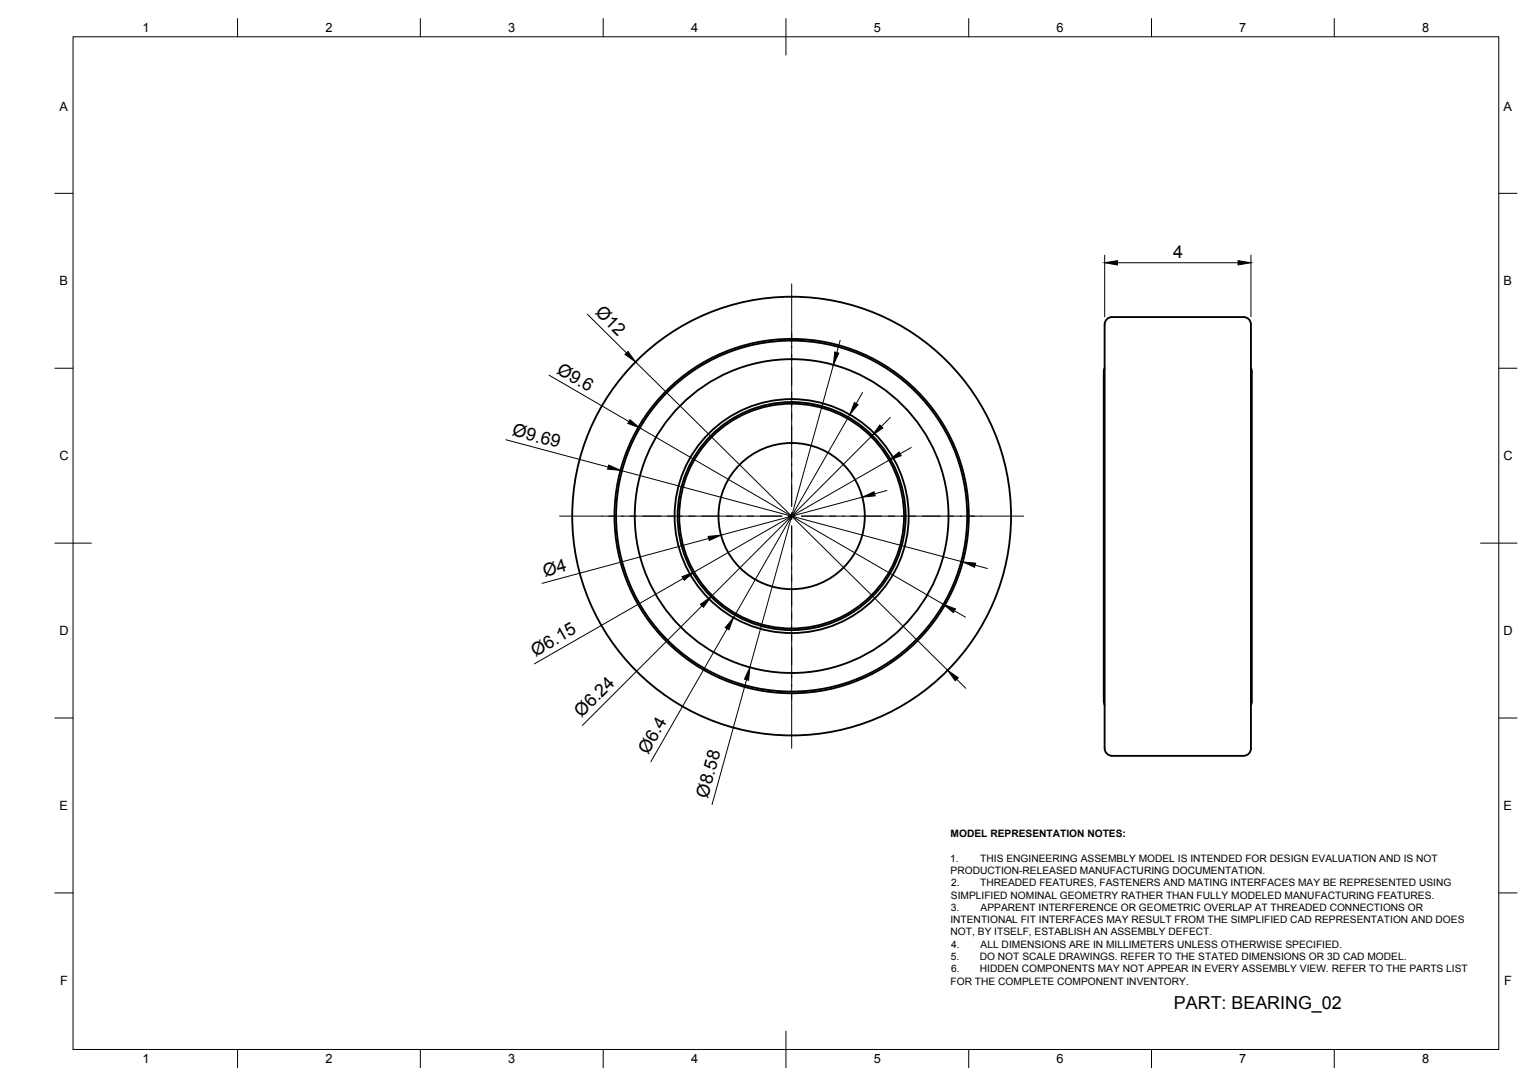
ISO-10303-21;
HEADER;
/* Generated by software containing ST-Developer
 * from STEP Tools, Inc. (www.steptools.com) 
 */

FILE_DESCRIPTION(
/* description */ (''),
/* implementation_level */ '2;1');

FILE_NAME(
/* name */ 'Bearing_02.step',
/* time_stamp */ '2026-10-04T15:18:51-07:00',
/* author */ (''),
/* organization */ (''),
/* preprocessor_version */ 'ST-DEVELOPER v20.2',
/* originating_system */ 'Autodesk Translation Framework v15.15.0.0',
/* authorisation */ '');

FILE_SCHEMA (('AUTOMOTIVE_DESIGN { 1 0 10303 214 3 1 1 }'));
ENDSEC;

DATA;
#10=MECHANICAL_DESIGN_GEOMETRIC_PRESENTATION_REPRESENTATION('',(#78,#79,#80,#81),#9891);
#59=SHAPE_REPRESENTATION_RELATIONSHIP('SRR','None',#9930,#67);
#67=ADVANCED_BREP_SHAPE_REPRESENTATION('',(#92,#93,#94,#95),#9890);
#78=STYLED_ITEM('',(#9972),#92);
#79=STYLED_ITEM('',(#9972),#93);
#80=STYLED_ITEM('',(#9972),#94);
#81=STYLED_ITEM('',(#9972),#95);
#92=MANIFOLD_SOLID_BREP('Body1',#5626);
#93=MANIFOLD_SOLID_BREP('Body2',#5627);
#94=MANIFOLD_SOLID_BREP('Body3',#5628);
#95=MANIFOLD_SOLID_BREP('Body4',#5629);
#143=FACE_BOUND('',#1063,.T.);
#144=FACE_BOUND('',#1065,.T.);
#145=FACE_BOUND('',#1067,.T.);
#146=FACE_BOUND('',#1069,.T.);
#147=FACE_BOUND('',#1081,.T.);
#148=FACE_BOUND('',#1083,.T.);
#149=FACE_BOUND('',#1085,.T.);
#150=FACE_BOUND('',#1087,.T.);
#151=FACE_BOUND('',#1101,.T.);
#152=FACE_BOUND('',#1103,.T.);
#153=FACE_BOUND('',#1105,.T.);
#154=FACE_BOUND('',#1107,.T.);
#155=FACE_BOUND('',#1109,.T.);
#156=FACE_BOUND('',#1123,.T.);
#157=FACE_BOUND('',#1125,.T.);
#158=FACE_BOUND('',#1127,.T.);
#159=FACE_BOUND('',#1129,.T.);
#160=FACE_BOUND('',#1131,.T.);
#319=PLANE('',#6244);
#320=PLANE('',#6245);
#321=PLANE('',#6246);
#322=PLANE('',#6247);
#323=PLANE('',#6277);
#324=PLANE('',#6278);
#325=PLANE('',#6279);
#326=PLANE('',#6280);
#327=PLANE('',#6317);
#328=PLANE('',#6318);
#329=PLANE('',#6319);
#330=PLANE('',#6320);
#331=PLANE('',#6321);
#332=PLANE('',#6358);
#333=PLANE('',#6359);
#334=PLANE('',#6360);
#335=PLANE('',#6361);
#336=PLANE('',#6362);
#360=TOROIDAL_SURFACE('',#6233,5.8,0.2);
#361=TOROIDAL_SURFACE('',#6239,5.8,0.2);
#362=TOROIDAL_SURFACE('',#6254,3.25741379310345,0.138976293103448);
#363=TOROIDAL_SURFACE('',#6260,3.25741379310345,0.138976293103448);
#364=TOROIDAL_SURFACE('',#6268,2.2,0.2);
#365=TOROIDAL_SURFACE('',#6274,2.2,0.2);
#366=TOROIDAL_SURFACE('',#6284,4.14313829631318,0.0900000000000005);
#367=TOROIDAL_SURFACE('',#6290,4.38370090847553,0.0200000000000002);
#368=TOROIDAL_SURFACE('',#6293,4.58,0.119999999999999);
#369=TOROIDAL_SURFACE('',#6299,4.51071796769724,0.12);
#370=TOROIDAL_SURFACE('',#6302,4.51071796769724,0.22);
#371=TOROIDAL_SURFACE('',#6308,4.58,0.219999999999999);
#372=TOROIDAL_SURFACE('',#6311,4.38370090847553,0.12);
#373=TOROIDAL_SURFACE('',#6325,4.14313829631318,0.0900000000000005);
#374=TOROIDAL_SURFACE('',#6331,4.38370090847553,0.0200000000000002);
#375=TOROIDAL_SURFACE('',#6334,4.58,0.119999999999999);
#376=TOROIDAL_SURFACE('',#6340,4.51071796769724,0.12);
#377=TOROIDAL_SURFACE('',#6343,4.51071796769724,0.22);
#378=TOROIDAL_SURFACE('',#6349,4.58,0.219999999999999);
#379=TOROIDAL_SURFACE('',#6352,4.38370090847553,0.12);
#395=CONICAL_SURFACE('',#6231,4.8,0.785398163397444);
#396=CONICAL_SURFACE('',#6242,4.845,0.785398163397444);
#397=CONICAL_SURFACE('',#6248,3.1184375,0.785398163397448);
#398=CONICAL_SURFACE('',#6266,3.0734375,0.785398163397448);
#399=CONICAL_SURFACE('',#6288,4.36638040039984,0.52359877559829);
#400=CONICAL_SURFACE('',#6297,4.57071796769724,1.04719755119659);
#401=CONICAL_SURFACE('',#6306,4.62071796769724,1.04719755119659);
#402=CONICAL_SURFACE('',#6315,4.27977786002139,0.52359877559829);
#403=CONICAL_SURFACE('',#6329,4.36638040039984,0.52359877559829);
#404=CONICAL_SURFACE('',#6338,4.57071796769724,1.04719755119659);
#405=CONICAL_SURFACE('',#6347,4.62071796769724,1.04719755119659);
#406=CONICAL_SURFACE('',#6356,4.27977786002139,0.52359877559829);
#677=FACE_OUTER_BOUND('',#1054,.T.);
#678=FACE_OUTER_BOUND('',#1055,.T.);
#679=FACE_OUTER_BOUND('',#1056,.T.);
#680=FACE_OUTER_BOUND('',#1057,.T.);
#681=FACE_OUTER_BOUND('',#1058,.T.);
#682=FACE_OUTER_BOUND('',#1059,.T.);
#683=FACE_OUTER_BOUND('',#1060,.T.);
#684=FACE_OUTER_BOUND('',#1061,.T.);
#685=FACE_OUTER_BOUND('',#1062,.T.);
#686=FACE_OUTER_BOUND('',#1064,.T.);
#687=FACE_OUTER_BOUND('',#1066,.T.);
#688=FACE_OUTER_BOUND('',#1068,.T.);
#689=FACE_OUTER_BOUND('',#1070,.T.);
#690=FACE_OUTER_BOUND('',#1071,.T.);
#691=FACE_OUTER_BOUND('',#1072,.T.);
#692=FACE_OUTER_BOUND('',#1073,.T.);
#693=FACE_OUTER_BOUND('',#1074,.T.);
#694=FACE_OUTER_BOUND('',#1075,.T.);
#695=FACE_OUTER_BOUND('',#1076,.T.);
#696=FACE_OUTER_BOUND('',#1077,.T.);
#697=FACE_OUTER_BOUND('',#1078,.T.);
#698=FACE_OUTER_BOUND('',#1079,.T.);
#699=FACE_OUTER_BOUND('',#1080,.T.);
#700=FACE_OUTER_BOUND('',#1082,.T.);
#701=FACE_OUTER_BOUND('',#1084,.T.);
#702=FACE_OUTER_BOUND('',#1086,.T.);
#703=FACE_OUTER_BOUND('',#1088,.T.);
#704=FACE_OUTER_BOUND('',#1089,.T.);
#705=FACE_OUTER_BOUND('',#1090,.T.);
#706=FACE_OUTER_BOUND('',#1091,.T.);
#707=FACE_OUTER_BOUND('',#1092,.T.);
#708=FACE_OUTER_BOUND('',#1093,.T.);
#709=FACE_OUTER_BOUND('',#1094,.T.);
#710=FACE_OUTER_BOUND('',#1095,.T.);
#711=FACE_OUTER_BOUND('',#1096,.T.);
#712=FACE_OUTER_BOUND('',#1097,.T.);
#713=FACE_OUTER_BOUND('',#1098,.T.);
#714=FACE_OUTER_BOUND('',#1099,.T.);
#715=FACE_OUTER_BOUND('',#1100,.T.);
#716=FACE_OUTER_BOUND('',#1102,.T.);
#717=FACE_OUTER_BOUND('',#1104,.T.);
#718=FACE_OUTER_BOUND('',#1106,.T.);
#719=FACE_OUTER_BOUND('',#1108,.T.);
#720=FACE_OUTER_BOUND('',#1110,.T.);
#721=FACE_OUTER_BOUND('',#1111,.T.);
#722=FACE_OUTER_BOUND('',#1112,.T.);
#723=FACE_OUTER_BOUND('',#1113,.T.);
#724=FACE_OUTER_BOUND('',#1114,.T.);
#725=FACE_OUTER_BOUND('',#1115,.T.);
#726=FACE_OUTER_BOUND('',#1116,.T.);
#727=FACE_OUTER_BOUND('',#1117,.T.);
#728=FACE_OUTER_BOUND('',#1118,.T.);
#729=FACE_OUTER_BOUND('',#1119,.T.);
#730=FACE_OUTER_BOUND('',#1120,.T.);
#731=FACE_OUTER_BOUND('',#1121,.T.);
#732=FACE_OUTER_BOUND('',#1122,.T.);
#733=FACE_OUTER_BOUND('',#1124,.T.);
#734=FACE_OUTER_BOUND('',#1126,.T.);
#735=FACE_OUTER_BOUND('',#1128,.T.);
#736=FACE_OUTER_BOUND('',#1130,.T.);
#1054=EDGE_LOOP('',(#4994,#4995,#4996,#4997));
#1055=EDGE_LOOP('',(#4998,#4999,#5000,#5001));
#1056=EDGE_LOOP('',(#5002,#5003,#5004,#5005,#5006));
#1057=EDGE_LOOP('',(#5007,#5008,#5009,#5010,#5011));
#1058=EDGE_LOOP('',(#5012,#5013,#5014,#5015));
#1059=EDGE_LOOP('',(#5016,#5017,#5018,#5019));
#1060=EDGE_LOOP('',(#5020,#5021,#5022,#5023));
#1061=EDGE_LOOP('',(#5024,#5025,#5026,#5027));
#1062=EDGE_LOOP('',(#5028));
#1063=EDGE_LOOP('',(#5029));
#1064=EDGE_LOOP('',(#5030));
#1065=EDGE_LOOP('',(#5031));
#1066=EDGE_LOOP('',(#5032));
#1067=EDGE_LOOP('',(#5033));
#1068=EDGE_LOOP('',(#5034));
#1069=EDGE_LOOP('',(#5035));
#1070=EDGE_LOOP('',(#5036,#5037,#5038,#5039,#5040));
#1071=EDGE_LOOP('',(#5041,#5042,#5043,#5044,#5045));
#1072=EDGE_LOOP('',(#5046,#5047,#5048,#5049));
#1073=EDGE_LOOP('',(#5050,#5051,#5052,#5053));
#1074=EDGE_LOOP('',(#5054,#5055,#5056,#5057));
#1075=EDGE_LOOP('',(#5058,#5059,#5060,#5061));
#1076=EDGE_LOOP('',(#5062,#5063,#5064,#5065));
#1077=EDGE_LOOP('',(#5066,#5067,#5068,#5069));
#1078=EDGE_LOOP('',(#5070,#5071,#5072,#5073));
#1079=EDGE_LOOP('',(#5074,#5075,#5076,#5077));
#1080=EDGE_LOOP('',(#5078));
#1081=EDGE_LOOP('',(#5079));
#1082=EDGE_LOOP('',(#5080));
#1083=EDGE_LOOP('',(#5081));
#1084=EDGE_LOOP('',(#5082));
#1085=EDGE_LOOP('',(#5083));
#1086=EDGE_LOOP('',(#5084));
#1087=EDGE_LOOP('',(#5085));
#1088=EDGE_LOOP('',(#5086,#5087,#5088,#5089));
#1089=EDGE_LOOP('',(#5090,#5091,#5092,#5093));
#1090=EDGE_LOOP('',(#5094,#5095,#5096,#5097));
#1091=EDGE_LOOP('',(#5098,#5099,#5100,#5101));
#1092=EDGE_LOOP('',(#5102,#5103,#5104,#5105));
#1093=EDGE_LOOP('',(#5106,#5107,#5108,#5109));
#1094=EDGE_LOOP('',(#5110,#5111,#5112,#5113));
#1095=EDGE_LOOP('',(#5114,#5115,#5116,#5117));
#1096=EDGE_LOOP('',(#5118,#5119,#5120,#5121));
#1097=EDGE_LOOP('',(#5122,#5123,#5124,#5125));
#1098=EDGE_LOOP('',(#5126,#5127,#5128,#5129));
#1099=EDGE_LOOP('',(#5130,#5131,#5132,#5133));
#1100=EDGE_LOOP('',(#5134));
#1101=EDGE_LOOP('',(#5135));
#1102=EDGE_LOOP('',(#5136));
#1103=EDGE_LOOP('',(#5137));
#1104=EDGE_LOOP('',(#5138));
#1105=EDGE_LOOP('',(#5139));
#1106=EDGE_LOOP('',(#5140));
#1107=EDGE_LOOP('',(#5141));
#1108=EDGE_LOOP('',(#5142));
#1109=EDGE_LOOP('',(#5143));
#1110=EDGE_LOOP('',(#5144,#5145,#5146,#5147));
#1111=EDGE_LOOP('',(#5148,#5149,#5150,#5151));
#1112=EDGE_LOOP('',(#5152,#5153,#5154,#5155));
#1113=EDGE_LOOP('',(#5156,#5157,#5158,#5159));
#1114=EDGE_LOOP('',(#5160,#5161,#5162,#5163));
#1115=EDGE_LOOP('',(#5164,#5165,#5166,#5167));
#1116=EDGE_LOOP('',(#5168,#5169,#5170,#5171));
#1117=EDGE_LOOP('',(#5172,#5173,#5174,#5175));
#1118=EDGE_LOOP('',(#5176,#5177,#5178,#5179));
#1119=EDGE_LOOP('',(#5180,#5181,#5182,#5183));
#1120=EDGE_LOOP('',(#5184,#5185,#5186,#5187));
#1121=EDGE_LOOP('',(#5188,#5189,#5190,#5191));
#1122=EDGE_LOOP('',(#5192));
#1123=EDGE_LOOP('',(#5193));
#1124=EDGE_LOOP('',(#5194));
#1125=EDGE_LOOP('',(#5195));
#1126=EDGE_LOOP('',(#5196));
#1127=EDGE_LOOP('',(#5197));
#1128=EDGE_LOOP('',(#5198));
#1129=EDGE_LOOP('',(#5199));
#1130=EDGE_LOOP('',(#5200));
#1131=EDGE_LOOP('',(#5201));
#1574=LINE('',#9642,#2038);
#1575=LINE('',#9648,#2039);
#1576=LINE('',#9656,#2040);
#1577=LINE('',#9660,#2041);
#1578=LINE('',#9671,#2042);
#1579=LINE('',#9678,#2043);
#1580=LINE('',#9689,#2044);
#1581=LINE('',#9694,#2045);
#1582=LINE('',#9704,#2046);
#1583=LINE('',#9714,#2047);
#1584=LINE('',#9718,#2048);
#1585=LINE('',#9728,#2049);
#1586=LINE('',#9742,#2050);
#1587=LINE('',#9753,#2051);
#1588=LINE('',#9767,#2052);
#1589=LINE('',#9781,#2053);
#1590=LINE('',#9795,#2054);
#1591=LINE('',#9805,#2055);
#1592=LINE('',#9816,#2056);
#1593=LINE('',#9830,#2057);
#1594=LINE('',#9844,#2058);
#1595=LINE('',#9858,#2059);
#2038=VECTOR('',#7821,4.8);
#2039=VECTOR('',#7828,4.872);
#2040=VECTOR('',#7837,4.8);
#2041=VECTOR('',#7842,4.8);
#2042=VECTOR('',#7857,6.);
#2043=VECTOR('',#7866,4.845);
#2044=VECTOR('',#7881,3.1184375);
#2045=VECTOR('',#7888,3.1184375);
#2046=VECTOR('',#7901,3.272);
#2047=VECTOR('',#7914,3.1184375);
#2048=VECTOR('',#7919,3.0734375);
#2049=VECTOR('',#7932,2.);
#2050=VECTOR('',#7953,3.2);
#2051=VECTOR('',#7968,4.36638040039984);
#2052=VECTOR('',#7987,4.57071796769724);
#2053=VECTOR('',#8006,4.62071796769724);
#2054=VECTOR('',#8025,4.27977786002139);
#2055=VECTOR('',#8040,3.2);
#2056=VECTOR('',#8055,4.36638040039984);
#2057=VECTOR('',#8074,4.57071796769724);
#2058=VECTOR('',#8093,4.62071796769724);
#2059=VECTOR('',#8112,4.27977786002139);
#2283=CIRCLE('',#6222,4.8);
#2284=CIRCLE('',#6223,4.8);
#2285=CIRCLE('',#6225,4.872);
#2286=CIRCLE('',#6226,4.872);
#2287=CIRCLE('',#6228,4.8);
#2288=CIRCLE('',#6229,4.8);
#2289=CIRCLE('',#6230,4.8);
#2290=CIRCLE('',#6232,4.845);
#2291=CIRCLE('',#6234,6.);
#2292=CIRCLE('',#6235,0.2);
#2293=CIRCLE('',#6236,5.8);
#2294=CIRCLE('',#6238,6.);
#2295=CIRCLE('',#6240,5.8);
#2296=CIRCLE('',#6241,0.2);
#2297=CIRCLE('',#6243,4.845);
#2298=CIRCLE('',#6249,3.1184375);
#2299=CIRCLE('',#6250,3.0734375);
#2300=CIRCLE('',#6251,3.1184375);
#2301=CIRCLE('',#6253,3.1184375);
#2302=CIRCLE('',#6255,0.138976293103448);
#2303=CIRCLE('',#6256,3.2);
#2304=CIRCLE('',#6258,3.272);
#2305=CIRCLE('',#6259,3.272);
#2306=CIRCLE('',#6261,3.2);
#2307=CIRCLE('',#6262,0.138976293103448);
#2308=CIRCLE('',#6263,3.1184375);
#2309=CIRCLE('',#6265,3.1184375);
#2310=CIRCLE('',#6267,3.0734375);
#2311=CIRCLE('',#6269,2.2);
#2312=CIRCLE('',#6270,0.2);
#2313=CIRCLE('',#6271,2.);
#2314=CIRCLE('',#6273,2.);
#2315=CIRCLE('',#6275,0.2);
#2316=CIRCLE('',#6276,2.2);
#2317=CIRCLE('',#6282,3.2);
#2318=CIRCLE('',#6283,3.2);
#2319=CIRCLE('',#6285,4.22108058265378);
#2320=CIRCLE('',#6286,0.0900000000000005);
#2321=CIRCLE('',#6287,4.14313829631318);
#2322=CIRCLE('',#6289,4.36638040039984);
#2323=CIRCLE('',#6291,4.38370090847553);
#2324=CIRCLE('',#6292,0.0200000000000002);
#2325=CIRCLE('',#6294,4.64);
#2326=CIRCLE('',#6295,0.119999999999999);
#2327=CIRCLE('',#6296,4.58);
#2328=CIRCLE('',#6298,4.57071796769724);
#2329=CIRCLE('',#6300,4.39071796769724);
#2330=CIRCLE('',#6301,0.12);
#2331=CIRCLE('',#6303,4.62071796769724);
#2332=CIRCLE('',#6304,0.22);
#2333=CIRCLE('',#6305,4.29071796769724);
#2334=CIRCLE('',#6307,4.69);
#2335=CIRCLE('',#6309,4.58);
#2336=CIRCLE('',#6310,0.219999999999999);
#2337=CIRCLE('',#6312,4.27977786002139);
#2338=CIRCLE('',#6313,0.12);
#2339=CIRCLE('',#6314,4.38370090847553);
#2340=CIRCLE('',#6316,4.13736479362129);
#2341=CIRCLE('',#6323,3.2);
#2342=CIRCLE('',#6324,3.2);
#2343=CIRCLE('',#6326,4.22108058265378);
#2344=CIRCLE('',#6327,0.0900000000000005);
#2345=CIRCLE('',#6328,4.14313829631318);
#2346=CIRCLE('',#6330,4.36638040039984);
#2347=CIRCLE('',#6332,4.38370090847553);
#2348=CIRCLE('',#6333,0.0200000000000002);
#2349=CIRCLE('',#6335,4.64);
#2350=CIRCLE('',#6336,0.119999999999999);
#2351=CIRCLE('',#6337,4.58);
#2352=CIRCLE('',#6339,4.57071796769724);
#2353=CIRCLE('',#6341,4.39071796769724);
#2354=CIRCLE('',#6342,0.12);
#2355=CIRCLE('',#6344,4.62071796769724);
#2356=CIRCLE('',#6345,0.22);
#2357=CIRCLE('',#6346,4.29071796769724);
#2358=CIRCLE('',#6348,4.69);
#2359=CIRCLE('',#6350,4.58);
#2360=CIRCLE('',#6351,0.219999999999999);
#2361=CIRCLE('',#6353,4.27977786002139);
#2362=CIRCLE('',#6354,0.12);
#2363=CIRCLE('',#6355,4.38370090847553);
#2364=CIRCLE('',#6357,4.13736479362129);
#2806=VERTEX_POINT('',#9639);
#2807=VERTEX_POINT('',#9641);
#2808=VERTEX_POINT('',#9645);
#2809=VERTEX_POINT('',#9647);
#2810=VERTEX_POINT('',#9651);
#2811=VERTEX_POINT('',#9652);
#2812=VERTEX_POINT('',#9655);
#2813=VERTEX_POINT('',#9659);
#2814=VERTEX_POINT('',#9663);
#2815=VERTEX_POINT('',#9665);
#2816=VERTEX_POINT('',#9669);
#2817=VERTEX_POINT('',#9673);
#2818=VERTEX_POINT('',#9677);
#2819=VERTEX_POINT('',#9685);
#2820=VERTEX_POINT('',#9686);
#2821=VERTEX_POINT('',#9688);
#2822=VERTEX_POINT('',#9693);
#2823=VERTEX_POINT('',#9697);
#2824=VERTEX_POINT('',#9701);
#2825=VERTEX_POINT('',#9703);
#2826=VERTEX_POINT('',#9707);
#2827=VERTEX_POINT('',#9709);
#2828=VERTEX_POINT('',#9713);
#2829=VERTEX_POINT('',#9717);
#2830=VERTEX_POINT('',#9721);
#2831=VERTEX_POINT('',#9723);
#2832=VERTEX_POINT('',#9727);
#2833=VERTEX_POINT('',#9731);
#2834=VERTEX_POINT('',#9739);
#2835=VERTEX_POINT('',#9741);
#2836=VERTEX_POINT('',#9745);
#2837=VERTEX_POINT('',#9747);
#2838=VERTEX_POINT('',#9751);
#2839=VERTEX_POINT('',#9755);
#2840=VERTEX_POINT('',#9759);
#2841=VERTEX_POINT('',#9761);
#2842=VERTEX_POINT('',#9765);
#2843=VERTEX_POINT('',#9769);
#2844=VERTEX_POINT('',#9773);
#2845=VERTEX_POINT('',#9775);
#2846=VERTEX_POINT('',#9779);
#2847=VERTEX_POINT('',#9783);
#2848=VERTEX_POINT('',#9787);
#2849=VERTEX_POINT('',#9789);
#2850=VERTEX_POINT('',#9793);
#2851=VERTEX_POINT('',#9802);
#2852=VERTEX_POINT('',#9804);
#2853=VERTEX_POINT('',#9808);
#2854=VERTEX_POINT('',#9810);
#2855=VERTEX_POINT('',#9814);
#2856=VERTEX_POINT('',#9818);
#2857=VERTEX_POINT('',#9822);
#2858=VERTEX_POINT('',#9824);
#2859=VERTEX_POINT('',#9828);
#2860=VERTEX_POINT('',#9832);
#2861=VERTEX_POINT('',#9836);
#2862=VERTEX_POINT('',#9838);
#2863=VERTEX_POINT('',#9842);
#2864=VERTEX_POINT('',#9846);
#2865=VERTEX_POINT('',#9850);
#2866=VERTEX_POINT('',#9852);
#2867=VERTEX_POINT('',#9856);
#3542=EDGE_CURVE('',#2806,#2806,#2283,.T.);
#3543=EDGE_CURVE('',#2806,#2807,#1574,.T.);
#3544=EDGE_CURVE('',#2807,#2807,#2284,.T.);
#3545=EDGE_CURVE('',#2808,#2808,#2285,.T.);
#3546=EDGE_CURVE('',#2808,#2809,#1575,.T.);
#3547=EDGE_CURVE('',#2809,#2809,#2286,.T.);
#3548=EDGE_CURVE('',#2810,#2811,#2287,.T.);
#3549=EDGE_CURVE('',#2811,#2810,#2288,.T.);
#3550=EDGE_CURVE('',#2811,#2812,#1576,.T.);
#3551=EDGE_CURVE('',#2812,#2812,#2289,.T.);
#3552=EDGE_CURVE('',#2810,#2813,#1577,.T.);
#3553=EDGE_CURVE('',#2813,#2813,#2290,.T.);
#3554=EDGE_CURVE('',#2814,#2814,#2291,.T.);
#3555=EDGE_CURVE('',#2814,#2815,#2292,.T.);
#3556=EDGE_CURVE('',#2815,#2815,#2293,.T.);
#3557=EDGE_CURVE('',#2816,#2816,#2294,.T.);
#3558=EDGE_CURVE('',#2816,#2814,#1578,.T.);
#3559=EDGE_CURVE('',#2817,#2817,#2295,.T.);
#3560=EDGE_CURVE('',#2817,#2816,#2296,.T.);
#3561=EDGE_CURVE('',#2807,#2818,#1579,.T.);
#3562=EDGE_CURVE('',#2818,#2818,#2297,.T.);
#3563=EDGE_CURVE('',#2819,#2820,#2298,.T.);
#3564=EDGE_CURVE('',#2820,#2821,#1580,.T.);
#3565=EDGE_CURVE('',#2821,#2821,#2299,.T.);
#3566=EDGE_CURVE('',#2820,#2819,#2300,.T.);
#3567=EDGE_CURVE('',#2819,#2822,#1581,.T.);
#3568=EDGE_CURVE('',#2822,#2822,#2301,.T.);
#3569=EDGE_CURVE('',#2822,#2823,#2302,.T.);
#3570=EDGE_CURVE('',#2823,#2823,#2303,.T.);
#3571=EDGE_CURVE('',#2824,#2824,#2304,.T.);
#3572=EDGE_CURVE('',#2824,#2825,#1582,.T.);
#3573=EDGE_CURVE('',#2825,#2825,#2305,.T.);
#3574=EDGE_CURVE('',#2826,#2826,#2306,.T.);
#3575=EDGE_CURVE('',#2826,#2827,#2307,.T.);
#3576=EDGE_CURVE('',#2827,#2827,#2308,.T.);
#3577=EDGE_CURVE('',#2827,#2828,#1583,.T.);
#3578=EDGE_CURVE('',#2828,#2828,#2309,.T.);
#3579=EDGE_CURVE('',#2828,#2829,#1584,.T.);
#3580=EDGE_CURVE('',#2829,#2829,#2310,.T.);
#3581=EDGE_CURVE('',#2830,#2830,#2311,.T.);
#3582=EDGE_CURVE('',#2830,#2831,#2312,.T.);
#3583=EDGE_CURVE('',#2831,#2831,#2313,.T.);
#3584=EDGE_CURVE('',#2831,#2832,#1585,.T.);
#3585=EDGE_CURVE('',#2832,#2832,#2314,.T.);
#3586=EDGE_CURVE('',#2832,#2833,#2315,.T.);
#3587=EDGE_CURVE('',#2833,#2833,#2316,.T.);
#3588=EDGE_CURVE('',#2834,#2834,#2317,.T.);
#3589=EDGE_CURVE('',#2834,#2835,#1586,.T.);
#3590=EDGE_CURVE('',#2835,#2835,#2318,.T.);
#3591=EDGE_CURVE('',#2836,#2836,#2319,.T.);
#3592=EDGE_CURVE('',#2836,#2837,#2320,.T.);
#3593=EDGE_CURVE('',#2837,#2837,#2321,.T.);
#3594=EDGE_CURVE('',#2838,#2838,#2322,.T.);
#3595=EDGE_CURVE('',#2838,#2836,#1587,.T.);
#3596=EDGE_CURVE('',#2839,#2839,#2323,.T.);
#3597=EDGE_CURVE('',#2839,#2838,#2324,.T.);
#3598=EDGE_CURVE('',#2840,#2840,#2325,.T.);
#3599=EDGE_CURVE('',#2840,#2841,#2326,.T.);
#3600=EDGE_CURVE('',#2841,#2841,#2327,.T.);
#3601=EDGE_CURVE('',#2842,#2842,#2328,.T.);
#3602=EDGE_CURVE('',#2842,#2840,#1588,.T.);
#3603=EDGE_CURVE('',#2843,#2843,#2329,.T.);
#3604=EDGE_CURVE('',#2843,#2842,#2330,.T.);
#3605=EDGE_CURVE('',#2844,#2844,#2331,.T.);
#3606=EDGE_CURVE('',#2844,#2845,#2332,.T.);
#3607=EDGE_CURVE('',#2845,#2845,#2333,.T.);
#3608=EDGE_CURVE('',#2846,#2846,#2334,.T.);
#3609=EDGE_CURVE('',#2846,#2844,#1589,.T.);
#3610=EDGE_CURVE('',#2847,#2847,#2335,.T.);
#3611=EDGE_CURVE('',#2847,#2846,#2336,.T.);
#3612=EDGE_CURVE('',#2848,#2848,#2337,.T.);
#3613=EDGE_CURVE('',#2848,#2849,#2338,.T.);
#3614=EDGE_CURVE('',#2849,#2849,#2339,.T.);
#3615=EDGE_CURVE('',#2850,#2850,#2340,.T.);
#3616=EDGE_CURVE('',#2850,#2848,#1590,.T.);
#3617=EDGE_CURVE('',#2851,#2851,#2341,.T.);
#3618=EDGE_CURVE('',#2851,#2852,#1591,.T.);
#3619=EDGE_CURVE('',#2852,#2852,#2342,.T.);
#3620=EDGE_CURVE('',#2853,#2853,#2343,.T.);
#3621=EDGE_CURVE('',#2853,#2854,#2344,.T.);
#3622=EDGE_CURVE('',#2854,#2854,#2345,.T.);
#3623=EDGE_CURVE('',#2855,#2855,#2346,.T.);
#3624=EDGE_CURVE('',#2855,#2853,#1592,.T.);
#3625=EDGE_CURVE('',#2856,#2856,#2347,.T.);
#3626=EDGE_CURVE('',#2856,#2855,#2348,.T.);
#3627=EDGE_CURVE('',#2857,#2857,#2349,.T.);
#3628=EDGE_CURVE('',#2857,#2858,#2350,.T.);
#3629=EDGE_CURVE('',#2858,#2858,#2351,.T.);
#3630=EDGE_CURVE('',#2859,#2859,#2352,.T.);
#3631=EDGE_CURVE('',#2859,#2857,#1593,.T.);
#3632=EDGE_CURVE('',#2860,#2860,#2353,.T.);
#3633=EDGE_CURVE('',#2860,#2859,#2354,.T.);
#3634=EDGE_CURVE('',#2861,#2861,#2355,.T.);
#3635=EDGE_CURVE('',#2861,#2862,#2356,.T.);
#3636=EDGE_CURVE('',#2862,#2862,#2357,.T.);
#3637=EDGE_CURVE('',#2863,#2863,#2358,.T.);
#3638=EDGE_CURVE('',#2863,#2861,#1594,.T.);
#3639=EDGE_CURVE('',#2864,#2864,#2359,.T.);
#3640=EDGE_CURVE('',#2864,#2863,#2360,.T.);
#3641=EDGE_CURVE('',#2865,#2865,#2361,.T.);
#3642=EDGE_CURVE('',#2865,#2866,#2362,.T.);
#3643=EDGE_CURVE('',#2866,#2866,#2363,.T.);
#3644=EDGE_CURVE('',#2867,#2867,#2364,.T.);
#3645=EDGE_CURVE('',#2867,#2865,#1595,.T.);
#4994=ORIENTED_EDGE('',*,*,#3542,.F.);
#4995=ORIENTED_EDGE('',*,*,#3543,.T.);
#4996=ORIENTED_EDGE('',*,*,#3544,.T.);
#4997=ORIENTED_EDGE('',*,*,#3543,.F.);
#4998=ORIENTED_EDGE('',*,*,#3545,.F.);
#4999=ORIENTED_EDGE('',*,*,#3546,.T.);
#5000=ORIENTED_EDGE('',*,*,#3547,.T.);
#5001=ORIENTED_EDGE('',*,*,#3546,.F.);
#5002=ORIENTED_EDGE('',*,*,#3548,.F.);
#5003=ORIENTED_EDGE('',*,*,#3549,.F.);
#5004=ORIENTED_EDGE('',*,*,#3550,.T.);
#5005=ORIENTED_EDGE('',*,*,#3551,.T.);
#5006=ORIENTED_EDGE('',*,*,#3550,.F.);
#5007=ORIENTED_EDGE('',*,*,#3548,.T.);
#5008=ORIENTED_EDGE('',*,*,#3549,.T.);
#5009=ORIENTED_EDGE('',*,*,#3552,.T.);
#5010=ORIENTED_EDGE('',*,*,#3553,.F.);
#5011=ORIENTED_EDGE('',*,*,#3552,.F.);
#5012=ORIENTED_EDGE('',*,*,#3554,.F.);
#5013=ORIENTED_EDGE('',*,*,#3555,.T.);
#5014=ORIENTED_EDGE('',*,*,#3556,.T.);
#5015=ORIENTED_EDGE('',*,*,#3555,.F.);
#5016=ORIENTED_EDGE('',*,*,#3557,.F.);
#5017=ORIENTED_EDGE('',*,*,#3558,.T.);
#5018=ORIENTED_EDGE('',*,*,#3554,.T.);
#5019=ORIENTED_EDGE('',*,*,#3558,.F.);
#5020=ORIENTED_EDGE('',*,*,#3559,.F.);
#5021=ORIENTED_EDGE('',*,*,#3560,.T.);
#5022=ORIENTED_EDGE('',*,*,#3557,.T.);
#5023=ORIENTED_EDGE('',*,*,#3560,.F.);
#5024=ORIENTED_EDGE('',*,*,#3544,.F.);
#5025=ORIENTED_EDGE('',*,*,#3561,.T.);
#5026=ORIENTED_EDGE('',*,*,#3562,.T.);
#5027=ORIENTED_EDGE('',*,*,#3561,.F.);
#5028=ORIENTED_EDGE('',*,*,#3559,.T.);
#5029=ORIENTED_EDGE('',*,*,#3562,.F.);
#5030=ORIENTED_EDGE('',*,*,#3556,.F.);
#5031=ORIENTED_EDGE('',*,*,#3553,.T.);
#5032=ORIENTED_EDGE('',*,*,#3545,.T.);
#5033=ORIENTED_EDGE('',*,*,#3551,.F.);
#5034=ORIENTED_EDGE('',*,*,#3547,.F.);
#5035=ORIENTED_EDGE('',*,*,#3542,.T.);
#5036=ORIENTED_EDGE('',*,*,#3563,.T.);
#5037=ORIENTED_EDGE('',*,*,#3564,.T.);
#5038=ORIENTED_EDGE('',*,*,#3565,.F.);
#5039=ORIENTED_EDGE('',*,*,#3564,.F.);
#5040=ORIENTED_EDGE('',*,*,#3566,.T.);
#5041=ORIENTED_EDGE('',*,*,#3563,.F.);
#5042=ORIENTED_EDGE('',*,*,#3567,.T.);
#5043=ORIENTED_EDGE('',*,*,#3568,.T.);
#5044=ORIENTED_EDGE('',*,*,#3567,.F.);
#5045=ORIENTED_EDGE('',*,*,#3566,.F.);
#5046=ORIENTED_EDGE('',*,*,#3568,.F.);
#5047=ORIENTED_EDGE('',*,*,#3569,.T.);
#5048=ORIENTED_EDGE('',*,*,#3570,.T.);
#5049=ORIENTED_EDGE('',*,*,#3569,.F.);
#5050=ORIENTED_EDGE('',*,*,#3571,.F.);
#5051=ORIENTED_EDGE('',*,*,#3572,.T.);
#5052=ORIENTED_EDGE('',*,*,#3573,.T.);
#5053=ORIENTED_EDGE('',*,*,#3572,.F.);
#5054=ORIENTED_EDGE('',*,*,#3574,.F.);
#5055=ORIENTED_EDGE('',*,*,#3575,.T.);
#5056=ORIENTED_EDGE('',*,*,#3576,.T.);
#5057=ORIENTED_EDGE('',*,*,#3575,.F.);
#5058=ORIENTED_EDGE('',*,*,#3576,.F.);
#5059=ORIENTED_EDGE('',*,*,#3577,.T.);
#5060=ORIENTED_EDGE('',*,*,#3578,.T.);
#5061=ORIENTED_EDGE('',*,*,#3577,.F.);
#5062=ORIENTED_EDGE('',*,*,#3578,.F.);
#5063=ORIENTED_EDGE('',*,*,#3579,.T.);
#5064=ORIENTED_EDGE('',*,*,#3580,.T.);
#5065=ORIENTED_EDGE('',*,*,#3579,.F.);
#5066=ORIENTED_EDGE('',*,*,#3581,.F.);
#5067=ORIENTED_EDGE('',*,*,#3582,.T.);
#5068=ORIENTED_EDGE('',*,*,#3583,.T.);
#5069=ORIENTED_EDGE('',*,*,#3582,.F.);
#5070=ORIENTED_EDGE('',*,*,#3583,.F.);
#5071=ORIENTED_EDGE('',*,*,#3584,.T.);
#5072=ORIENTED_EDGE('',*,*,#3585,.T.);
#5073=ORIENTED_EDGE('',*,*,#3584,.F.);
#5074=ORIENTED_EDGE('',*,*,#3585,.F.);
#5075=ORIENTED_EDGE('',*,*,#3586,.T.);
#5076=ORIENTED_EDGE('',*,*,#3587,.T.);
#5077=ORIENTED_EDGE('',*,*,#3586,.F.);
#5078=ORIENTED_EDGE('',*,*,#3580,.F.);
#5079=ORIENTED_EDGE('',*,*,#3581,.T.);
#5080=ORIENTED_EDGE('',*,*,#3573,.F.);
#5081=ORIENTED_EDGE('',*,*,#3574,.T.);
#5082=ORIENTED_EDGE('',*,*,#3571,.T.);
#5083=ORIENTED_EDGE('',*,*,#3570,.F.);
#5084=ORIENTED_EDGE('',*,*,#3565,.T.);
#5085=ORIENTED_EDGE('',*,*,#3587,.F.);
#5086=ORIENTED_EDGE('',*,*,#3588,.F.);
#5087=ORIENTED_EDGE('',*,*,#3589,.T.);
#5088=ORIENTED_EDGE('',*,*,#3590,.T.);
#5089=ORIENTED_EDGE('',*,*,#3589,.F.);
#5090=ORIENTED_EDGE('',*,*,#3591,.F.);
#5091=ORIENTED_EDGE('',*,*,#3592,.T.);
#5092=ORIENTED_EDGE('',*,*,#3593,.T.);
#5093=ORIENTED_EDGE('',*,*,#3592,.F.);
#5094=ORIENTED_EDGE('',*,*,#3594,.F.);
#5095=ORIENTED_EDGE('',*,*,#3595,.T.);
#5096=ORIENTED_EDGE('',*,*,#3591,.T.);
#5097=ORIENTED_EDGE('',*,*,#3595,.F.);
#5098=ORIENTED_EDGE('',*,*,#3596,.F.);
#5099=ORIENTED_EDGE('',*,*,#3597,.T.);
#5100=ORIENTED_EDGE('',*,*,#3594,.T.);
#5101=ORIENTED_EDGE('',*,*,#3597,.F.);
#5102=ORIENTED_EDGE('',*,*,#3598,.F.);
#5103=ORIENTED_EDGE('',*,*,#3599,.T.);
#5104=ORIENTED_EDGE('',*,*,#3600,.T.);
#5105=ORIENTED_EDGE('',*,*,#3599,.F.);
#5106=ORIENTED_EDGE('',*,*,#3601,.F.);
#5107=ORIENTED_EDGE('',*,*,#3602,.T.);
#5108=ORIENTED_EDGE('',*,*,#3598,.T.);
#5109=ORIENTED_EDGE('',*,*,#3602,.F.);
#5110=ORIENTED_EDGE('',*,*,#3603,.F.);
#5111=ORIENTED_EDGE('',*,*,#3604,.T.);
#5112=ORIENTED_EDGE('',*,*,#3601,.T.);
#5113=ORIENTED_EDGE('',*,*,#3604,.F.);
#5114=ORIENTED_EDGE('',*,*,#3605,.F.);
#5115=ORIENTED_EDGE('',*,*,#3606,.T.);
#5116=ORIENTED_EDGE('',*,*,#3607,.T.);
#5117=ORIENTED_EDGE('',*,*,#3606,.F.);
#5118=ORIENTED_EDGE('',*,*,#3608,.F.);
#5119=ORIENTED_EDGE('',*,*,#3609,.T.);
#5120=ORIENTED_EDGE('',*,*,#3605,.T.);
#5121=ORIENTED_EDGE('',*,*,#3609,.F.);
#5122=ORIENTED_EDGE('',*,*,#3610,.F.);
#5123=ORIENTED_EDGE('',*,*,#3611,.T.);
#5124=ORIENTED_EDGE('',*,*,#3608,.T.);
#5125=ORIENTED_EDGE('',*,*,#3611,.F.);
#5126=ORIENTED_EDGE('',*,*,#3612,.F.);
#5127=ORIENTED_EDGE('',*,*,#3613,.T.);
#5128=ORIENTED_EDGE('',*,*,#3614,.T.);
#5129=ORIENTED_EDGE('',*,*,#3613,.F.);
#5130=ORIENTED_EDGE('',*,*,#3615,.F.);
#5131=ORIENTED_EDGE('',*,*,#3616,.T.);
#5132=ORIENTED_EDGE('',*,*,#3612,.T.);
#5133=ORIENTED_EDGE('',*,*,#3616,.F.);
#5134=ORIENTED_EDGE('',*,*,#3615,.T.);
#5135=ORIENTED_EDGE('',*,*,#3590,.F.);
#5136=ORIENTED_EDGE('',*,*,#3610,.T.);
#5137=ORIENTED_EDGE('',*,*,#3614,.F.);
#5138=ORIENTED_EDGE('',*,*,#3603,.T.);
#5139=ORIENTED_EDGE('',*,*,#3607,.F.);
#5140=ORIENTED_EDGE('',*,*,#3600,.F.);
#5141=ORIENTED_EDGE('',*,*,#3596,.T.);
#5142=ORIENTED_EDGE('',*,*,#3593,.F.);
#5143=ORIENTED_EDGE('',*,*,#3588,.T.);
#5144=ORIENTED_EDGE('',*,*,#3617,.T.);
#5145=ORIENTED_EDGE('',*,*,#3618,.T.);
#5146=ORIENTED_EDGE('',*,*,#3619,.F.);
#5147=ORIENTED_EDGE('',*,*,#3618,.F.);
#5148=ORIENTED_EDGE('',*,*,#3620,.T.);
#5149=ORIENTED_EDGE('',*,*,#3621,.T.);
#5150=ORIENTED_EDGE('',*,*,#3622,.F.);
#5151=ORIENTED_EDGE('',*,*,#3621,.F.);
#5152=ORIENTED_EDGE('',*,*,#3623,.T.);
#5153=ORIENTED_EDGE('',*,*,#3624,.T.);
#5154=ORIENTED_EDGE('',*,*,#3620,.F.);
#5155=ORIENTED_EDGE('',*,*,#3624,.F.);
#5156=ORIENTED_EDGE('',*,*,#3625,.T.);
#5157=ORIENTED_EDGE('',*,*,#3626,.T.);
#5158=ORIENTED_EDGE('',*,*,#3623,.F.);
#5159=ORIENTED_EDGE('',*,*,#3626,.F.);
#5160=ORIENTED_EDGE('',*,*,#3627,.T.);
#5161=ORIENTED_EDGE('',*,*,#3628,.T.);
#5162=ORIENTED_EDGE('',*,*,#3629,.F.);
#5163=ORIENTED_EDGE('',*,*,#3628,.F.);
#5164=ORIENTED_EDGE('',*,*,#3630,.T.);
#5165=ORIENTED_EDGE('',*,*,#3631,.T.);
#5166=ORIENTED_EDGE('',*,*,#3627,.F.);
#5167=ORIENTED_EDGE('',*,*,#3631,.F.);
#5168=ORIENTED_EDGE('',*,*,#3632,.T.);
#5169=ORIENTED_EDGE('',*,*,#3633,.T.);
#5170=ORIENTED_EDGE('',*,*,#3630,.F.);
#5171=ORIENTED_EDGE('',*,*,#3633,.F.);
#5172=ORIENTED_EDGE('',*,*,#3634,.T.);
#5173=ORIENTED_EDGE('',*,*,#3635,.T.);
#5174=ORIENTED_EDGE('',*,*,#3636,.F.);
#5175=ORIENTED_EDGE('',*,*,#3635,.F.);
#5176=ORIENTED_EDGE('',*,*,#3637,.T.);
#5177=ORIENTED_EDGE('',*,*,#3638,.T.);
#5178=ORIENTED_EDGE('',*,*,#3634,.F.);
#5179=ORIENTED_EDGE('',*,*,#3638,.F.);
#5180=ORIENTED_EDGE('',*,*,#3639,.T.);
#5181=ORIENTED_EDGE('',*,*,#3640,.T.);
#5182=ORIENTED_EDGE('',*,*,#3637,.F.);
#5183=ORIENTED_EDGE('',*,*,#3640,.F.);
#5184=ORIENTED_EDGE('',*,*,#3641,.T.);
#5185=ORIENTED_EDGE('',*,*,#3642,.T.);
#5186=ORIENTED_EDGE('',*,*,#3643,.F.);
#5187=ORIENTED_EDGE('',*,*,#3642,.F.);
#5188=ORIENTED_EDGE('',*,*,#3644,.T.);
#5189=ORIENTED_EDGE('',*,*,#3645,.T.);
#5190=ORIENTED_EDGE('',*,*,#3641,.F.);
#5191=ORIENTED_EDGE('',*,*,#3645,.F.);
#5192=ORIENTED_EDGE('',*,*,#3644,.F.);
#5193=ORIENTED_EDGE('',*,*,#3619,.T.);
#5194=ORIENTED_EDGE('',*,*,#3639,.F.);
#5195=ORIENTED_EDGE('',*,*,#3643,.T.);
#5196=ORIENTED_EDGE('',*,*,#3632,.F.);
#5197=ORIENTED_EDGE('',*,*,#3636,.T.);
#5198=ORIENTED_EDGE('',*,*,#3629,.T.);
#5199=ORIENTED_EDGE('',*,*,#3625,.F.);
#5200=ORIENTED_EDGE('',*,*,#3622,.T.);
#5201=ORIENTED_EDGE('',*,*,#3617,.F.);
#5276=CYLINDRICAL_SURFACE('',#6221,4.8);
#5277=CYLINDRICAL_SURFACE('',#6224,4.872);
#5278=CYLINDRICAL_SURFACE('',#6227,4.8);
#5279=CYLINDRICAL_SURFACE('',#6237,6.);
#5280=CYLINDRICAL_SURFACE('',#6252,3.1184375);
#5281=CYLINDRICAL_SURFACE('',#6257,3.272);
#5282=CYLINDRICAL_SURFACE('',#6264,3.1184375);
#5283=CYLINDRICAL_SURFACE('',#6272,2.);
#5284=CYLINDRICAL_SURFACE('',#6281,3.2);
#5285=CYLINDRICAL_SURFACE('',#6322,3.2);
#5556=ADVANCED_FACE('',(#677),#5276,.F.);
#5557=ADVANCED_FACE('',(#678),#5277,.F.);
#5558=ADVANCED_FACE('',(#679),#5278,.F.);
#5559=ADVANCED_FACE('',(#680),#395,.F.);
#5560=ADVANCED_FACE('',(#681),#360,.T.);
#5561=ADVANCED_FACE('',(#682),#5279,.T.);
#5562=ADVANCED_FACE('',(#683),#361,.T.);
#5563=ADVANCED_FACE('',(#684),#396,.F.);
#5564=ADVANCED_FACE('',(#685,#143),#319,.F.);
#5565=ADVANCED_FACE('',(#686,#144),#320,.F.);
#5566=ADVANCED_FACE('',(#687,#145),#321,.F.);
#5567=ADVANCED_FACE('',(#688,#146),#322,.F.);
#5568=ADVANCED_FACE('',(#689),#397,.T.);
#5569=ADVANCED_FACE('',(#690),#5280,.T.);
#5570=ADVANCED_FACE('',(#691),#362,.F.);
#5571=ADVANCED_FACE('',(#692),#5281,.T.);
#5572=ADVANCED_FACE('',(#693),#363,.F.);
#5573=ADVANCED_FACE('',(#694),#5282,.T.);
#5574=ADVANCED_FACE('',(#695),#398,.T.);
#5575=ADVANCED_FACE('',(#696),#364,.T.);
#5576=ADVANCED_FACE('',(#697),#5283,.F.);
#5577=ADVANCED_FACE('',(#698),#365,.T.);
#5578=ADVANCED_FACE('',(#699,#147),#323,.F.);
#5579=ADVANCED_FACE('',(#700,#148),#324,.F.);
#5580=ADVANCED_FACE('',(#701,#149),#325,.F.);
#5581=ADVANCED_FACE('',(#702,#150),#326,.F.);
#5582=ADVANCED_FACE('',(#703),#5284,.F.);
#5583=ADVANCED_FACE('',(#704),#366,.T.);
#5584=ADVANCED_FACE('',(#705),#399,.T.);
#5585=ADVANCED_FACE('',(#706),#367,.F.);
#5586=ADVANCED_FACE('',(#707),#368,.F.);
#5587=ADVANCED_FACE('',(#708),#400,.F.);
#5588=ADVANCED_FACE('',(#709),#369,.F.);
#5589=ADVANCED_FACE('',(#710),#370,.T.);
#5590=ADVANCED_FACE('',(#711),#401,.T.);
#5591=ADVANCED_FACE('',(#712),#371,.T.);
#5592=ADVANCED_FACE('',(#713),#372,.T.);
#5593=ADVANCED_FACE('',(#714),#402,.F.);
#5594=ADVANCED_FACE('',(#715,#151),#327,.F.);
#5595=ADVANCED_FACE('',(#716,#152),#328,.F.);
#5596=ADVANCED_FACE('',(#717,#153),#329,.T.);
#5597=ADVANCED_FACE('',(#718,#154),#330,.T.);
#5598=ADVANCED_FACE('',(#719,#155),#331,.T.);
#5599=ADVANCED_FACE('',(#720),#5285,.F.);
#5600=ADVANCED_FACE('',(#721),#373,.T.);
#5601=ADVANCED_FACE('',(#722),#403,.T.);
#5602=ADVANCED_FACE('',(#723),#374,.F.);
#5603=ADVANCED_FACE('',(#724),#375,.F.);
#5604=ADVANCED_FACE('',(#725),#404,.F.);
#5605=ADVANCED_FACE('',(#726),#376,.F.);
#5606=ADVANCED_FACE('',(#727),#377,.T.);
#5607=ADVANCED_FACE('',(#728),#405,.T.);
#5608=ADVANCED_FACE('',(#729),#378,.T.);
#5609=ADVANCED_FACE('',(#730),#379,.T.);
#5610=ADVANCED_FACE('',(#731),#406,.F.);
#5611=ADVANCED_FACE('',(#732,#156),#332,.F.);
#5612=ADVANCED_FACE('',(#733,#157),#333,.F.);
#5613=ADVANCED_FACE('',(#734,#158),#334,.T.);
#5614=ADVANCED_FACE('',(#735,#159),#335,.T.);
#5615=ADVANCED_FACE('',(#736,#160),#336,.T.);
#5626=CLOSED_SHELL('',(#5556,#5557,#5558,#5559,#5560,#5561,#5562,#5563,
#5564,#5565,#5566,#5567));
#5627=CLOSED_SHELL('',(#5568,#5569,#5570,#5571,#5572,#5573,#5574,#5575,
#5576,#5577,#5578,#5579,#5580,#5581));
#5628=CLOSED_SHELL('',(#5582,#5583,#5584,#5585,#5586,#5587,#5588,#5589,
#5590,#5591,#5592,#5593,#5594,#5595,#5596,#5597,#5598));
#5629=CLOSED_SHELL('',(#5599,#5600,#5601,#5602,#5603,#5604,#5605,#5606,
#5607,#5608,#5609,#5610,#5611,#5612,#5613,#5614,#5615));
#6220=AXIS2_PLACEMENT_3D('',#9637,#7815,#7816);
#6221=AXIS2_PLACEMENT_3D('',#9638,#7817,#7818);
#6222=AXIS2_PLACEMENT_3D('',#9640,#7819,#7820);
#6223=AXIS2_PLACEMENT_3D('',#9643,#7822,#7823);
#6224=AXIS2_PLACEMENT_3D('',#9644,#7824,#7825);
#6225=AXIS2_PLACEMENT_3D('',#9646,#7826,#7827);
#6226=AXIS2_PLACEMENT_3D('',#9649,#7829,#7830);
#6227=AXIS2_PLACEMENT_3D('',#9650,#7831,#7832);
#6228=AXIS2_PLACEMENT_3D('',#9653,#7833,#7834);
#6229=AXIS2_PLACEMENT_3D('',#9654,#7835,#7836);
#6230=AXIS2_PLACEMENT_3D('',#9657,#7838,#7839);
#6231=AXIS2_PLACEMENT_3D('',#9658,#7840,#7841);
#6232=AXIS2_PLACEMENT_3D('',#9661,#7843,#7844);
#6233=AXIS2_PLACEMENT_3D('',#9662,#7845,#7846);
#6234=AXIS2_PLACEMENT_3D('',#9664,#7847,#7848);
#6235=AXIS2_PLACEMENT_3D('',#9666,#7849,#7850);
#6236=AXIS2_PLACEMENT_3D('',#9667,#7851,#7852);
#6237=AXIS2_PLACEMENT_3D('',#9668,#7853,#7854);
#6238=AXIS2_PLACEMENT_3D('',#9670,#7855,#7856);
#6239=AXIS2_PLACEMENT_3D('',#9672,#7858,#7859);
#6240=AXIS2_PLACEMENT_3D('',#9674,#7860,#7861);
#6241=AXIS2_PLACEMENT_3D('',#9675,#7862,#7863);
#6242=AXIS2_PLACEMENT_3D('',#9676,#7864,#7865);
#6243=AXIS2_PLACEMENT_3D('',#9679,#7867,#7868);
#6244=AXIS2_PLACEMENT_3D('',#9680,#7869,#7870);
#6245=AXIS2_PLACEMENT_3D('',#9681,#7871,#7872);
#6246=AXIS2_PLACEMENT_3D('',#9682,#7873,#7874);
#6247=AXIS2_PLACEMENT_3D('',#9683,#7875,#7876);
#6248=AXIS2_PLACEMENT_3D('',#9684,#7877,#7878);
#6249=AXIS2_PLACEMENT_3D('',#9687,#7879,#7880);
#6250=AXIS2_PLACEMENT_3D('',#9690,#7882,#7883);
#6251=AXIS2_PLACEMENT_3D('',#9691,#7884,#7885);
#6252=AXIS2_PLACEMENT_3D('',#9692,#7886,#7887);
#6253=AXIS2_PLACEMENT_3D('',#9695,#7889,#7890);
#6254=AXIS2_PLACEMENT_3D('',#9696,#7891,#7892);
#6255=AXIS2_PLACEMENT_3D('',#9698,#7893,#7894);
#6256=AXIS2_PLACEMENT_3D('',#9699,#7895,#7896);
#6257=AXIS2_PLACEMENT_3D('',#9700,#7897,#7898);
#6258=AXIS2_PLACEMENT_3D('',#9702,#7899,#7900);
#6259=AXIS2_PLACEMENT_3D('',#9705,#7902,#7903);
#6260=AXIS2_PLACEMENT_3D('',#9706,#7904,#7905);
#6261=AXIS2_PLACEMENT_3D('',#9708,#7906,#7907);
#6262=AXIS2_PLACEMENT_3D('',#9710,#7908,#7909);
#6263=AXIS2_PLACEMENT_3D('',#9711,#7910,#7911);
#6264=AXIS2_PLACEMENT_3D('',#9712,#7912,#7913);
#6265=AXIS2_PLACEMENT_3D('',#9715,#7915,#7916);
#6266=AXIS2_PLACEMENT_3D('',#9716,#7917,#7918);
#6267=AXIS2_PLACEMENT_3D('',#9719,#7920,#7921);
#6268=AXIS2_PLACEMENT_3D('',#9720,#7922,#7923);
#6269=AXIS2_PLACEMENT_3D('',#9722,#7924,#7925);
#6270=AXIS2_PLACEMENT_3D('',#9724,#7926,#7927);
#6271=AXIS2_PLACEMENT_3D('',#9725,#7928,#7929);
#6272=AXIS2_PLACEMENT_3D('',#9726,#7930,#7931);
#6273=AXIS2_PLACEMENT_3D('',#9729,#7933,#7934);
#6274=AXIS2_PLACEMENT_3D('',#9730,#7935,#7936);
#6275=AXIS2_PLACEMENT_3D('',#9732,#7937,#7938);
#6276=AXIS2_PLACEMENT_3D('',#9733,#7939,#7940);
#6277=AXIS2_PLACEMENT_3D('',#9734,#7941,#7942);
#6278=AXIS2_PLACEMENT_3D('',#9735,#7943,#7944);
#6279=AXIS2_PLACEMENT_3D('',#9736,#7945,#7946);
#6280=AXIS2_PLACEMENT_3D('',#9737,#7947,#7948);
#6281=AXIS2_PLACEMENT_3D('',#9738,#7949,#7950);
#6282=AXIS2_PLACEMENT_3D('',#9740,#7951,#7952);
#6283=AXIS2_PLACEMENT_3D('',#9743,#7954,#7955);
#6284=AXIS2_PLACEMENT_3D('',#9744,#7956,#7957);
#6285=AXIS2_PLACEMENT_3D('',#9746,#7958,#7959);
#6286=AXIS2_PLACEMENT_3D('',#9748,#7960,#7961);
#6287=AXIS2_PLACEMENT_3D('',#9749,#7962,#7963);
#6288=AXIS2_PLACEMENT_3D('',#9750,#7964,#7965);
#6289=AXIS2_PLACEMENT_3D('',#9752,#7966,#7967);
#6290=AXIS2_PLACEMENT_3D('',#9754,#7969,#7970);
#6291=AXIS2_PLACEMENT_3D('',#9756,#7971,#7972);
#6292=AXIS2_PLACEMENT_3D('',#9757,#7973,#7974);
#6293=AXIS2_PLACEMENT_3D('',#9758,#7975,#7976);
#6294=AXIS2_PLACEMENT_3D('',#9760,#7977,#7978);
#6295=AXIS2_PLACEMENT_3D('',#9762,#7979,#7980);
#6296=AXIS2_PLACEMENT_3D('',#9763,#7981,#7982);
#6297=AXIS2_PLACEMENT_3D('',#9764,#7983,#7984);
#6298=AXIS2_PLACEMENT_3D('',#9766,#7985,#7986);
#6299=AXIS2_PLACEMENT_3D('',#9768,#7988,#7989);
#6300=AXIS2_PLACEMENT_3D('',#9770,#7990,#7991);
#6301=AXIS2_PLACEMENT_3D('',#9771,#7992,#7993);
#6302=AXIS2_PLACEMENT_3D('',#9772,#7994,#7995);
#6303=AXIS2_PLACEMENT_3D('',#9774,#7996,#7997);
#6304=AXIS2_PLACEMENT_3D('',#9776,#7998,#7999);
#6305=AXIS2_PLACEMENT_3D('',#9777,#8000,#8001);
#6306=AXIS2_PLACEMENT_3D('',#9778,#8002,#8003);
#6307=AXIS2_PLACEMENT_3D('',#9780,#8004,#8005);
#6308=AXIS2_PLACEMENT_3D('',#9782,#8007,#8008);
#6309=AXIS2_PLACEMENT_3D('',#9784,#8009,#8010);
#6310=AXIS2_PLACEMENT_3D('',#9785,#8011,#8012);
#6311=AXIS2_PLACEMENT_3D('',#9786,#8013,#8014);
#6312=AXIS2_PLACEMENT_3D('',#9788,#8015,#8016);
#6313=AXIS2_PLACEMENT_3D('',#9790,#8017,#8018);
#6314=AXIS2_PLACEMENT_3D('',#9791,#8019,#8020);
#6315=AXIS2_PLACEMENT_3D('',#9792,#8021,#8022);
#6316=AXIS2_PLACEMENT_3D('',#9794,#8023,#8024);
#6317=AXIS2_PLACEMENT_3D('',#9796,#8026,#8027);
#6318=AXIS2_PLACEMENT_3D('',#9797,#8028,#8029);
#6319=AXIS2_PLACEMENT_3D('',#9798,#8030,#8031);
#6320=AXIS2_PLACEMENT_3D('',#9799,#8032,#8033);
#6321=AXIS2_PLACEMENT_3D('',#9800,#8034,#8035);
#6322=AXIS2_PLACEMENT_3D('',#9801,#8036,#8037);
#6323=AXIS2_PLACEMENT_3D('',#9803,#8038,#8039);
#6324=AXIS2_PLACEMENT_3D('',#9806,#8041,#8042);
#6325=AXIS2_PLACEMENT_3D('',#9807,#8043,#8044);
#6326=AXIS2_PLACEMENT_3D('',#9809,#8045,#8046);
#6327=AXIS2_PLACEMENT_3D('',#9811,#8047,#8048);
#6328=AXIS2_PLACEMENT_3D('',#9812,#8049,#8050);
#6329=AXIS2_PLACEMENT_3D('',#9813,#8051,#8052);
#6330=AXIS2_PLACEMENT_3D('',#9815,#8053,#8054);
#6331=AXIS2_PLACEMENT_3D('',#9817,#8056,#8057);
#6332=AXIS2_PLACEMENT_3D('',#9819,#8058,#8059);
#6333=AXIS2_PLACEMENT_3D('',#9820,#8060,#8061);
#6334=AXIS2_PLACEMENT_3D('',#9821,#8062,#8063);
#6335=AXIS2_PLACEMENT_3D('',#9823,#8064,#8065);
#6336=AXIS2_PLACEMENT_3D('',#9825,#8066,#8067);
#6337=AXIS2_PLACEMENT_3D('',#9826,#8068,#8069);
#6338=AXIS2_PLACEMENT_3D('',#9827,#8070,#8071);
#6339=AXIS2_PLACEMENT_3D('',#9829,#8072,#8073);
#6340=AXIS2_PLACEMENT_3D('',#9831,#8075,#8076);
#6341=AXIS2_PLACEMENT_3D('',#9833,#8077,#8078);
#6342=AXIS2_PLACEMENT_3D('',#9834,#8079,#8080);
#6343=AXIS2_PLACEMENT_3D('',#9835,#8081,#8082);
#6344=AXIS2_PLACEMENT_3D('',#9837,#8083,#8084);
#6345=AXIS2_PLACEMENT_3D('',#9839,#8085,#8086);
#6346=AXIS2_PLACEMENT_3D('',#9840,#8087,#8088);
#6347=AXIS2_PLACEMENT_3D('',#9841,#8089,#8090);
#6348=AXIS2_PLACEMENT_3D('',#9843,#8091,#8092);
#6349=AXIS2_PLACEMENT_3D('',#9845,#8094,#8095);
#6350=AXIS2_PLACEMENT_3D('',#9847,#8096,#8097);
#6351=AXIS2_PLACEMENT_3D('',#9848,#8098,#8099);
#6352=AXIS2_PLACEMENT_3D('',#9849,#8100,#8101);
#6353=AXIS2_PLACEMENT_3D('',#9851,#8102,#8103);
#6354=AXIS2_PLACEMENT_3D('',#9853,#8104,#8105);
#6355=AXIS2_PLACEMENT_3D('',#9854,#8106,#8107);
#6356=AXIS2_PLACEMENT_3D('',#9855,#8108,#8109);
#6357=AXIS2_PLACEMENT_3D('',#9857,#8110,#8111);
#6358=AXIS2_PLACEMENT_3D('',#9859,#8113,#8114);
#6359=AXIS2_PLACEMENT_3D('',#9860,#8115,#8116);
#6360=AXIS2_PLACEMENT_3D('',#9861,#8117,#8118);
#6361=AXIS2_PLACEMENT_3D('',#9862,#8119,#8120);
#6362=AXIS2_PLACEMENT_3D('',#9863,#8121,#8122);
#7815=DIRECTION('axis',(0.,0.,1.));
#7816=DIRECTION('refdir',(1.,0.,0.));
#7817=DIRECTION('center_axis',(-1.,-1.83697019872103E-16,0.));
#7818=DIRECTION('ref_axis',(1.83697019872103E-16,-1.,0.));
#7819=DIRECTION('center_axis',(-1.,-1.83697019872103E-16,0.));
#7820=DIRECTION('ref_axis',(1.83697019872103E-16,-1.,0.));
#7821=DIRECTION('',(-1.,-1.83697019872103E-16,0.));
#7822=DIRECTION('center_axis',(-1.,-1.83697019872103E-16,0.));
#7823=DIRECTION('ref_axis',(1.83697019872103E-16,-1.,0.));
#7824=DIRECTION('center_axis',(-1.,-1.83697019872103E-16,0.));
#7825=DIRECTION('ref_axis',(1.83697019872103E-16,-1.,0.));
#7826=DIRECTION('center_axis',(-1.,-1.83697019872103E-16,0.));
#7827=DIRECTION('ref_axis',(1.83697019872103E-16,-1.,0.));
#7828=DIRECTION('',(-1.,-1.83697019872103E-16,0.));
#7829=DIRECTION('center_axis',(-1.,-1.83697019872103E-16,0.));
#7830=DIRECTION('ref_axis',(1.83697019872103E-16,-1.,0.));
#7831=DIRECTION('center_axis',(-1.,-1.83697019872103E-16,0.));
#7832=DIRECTION('ref_axis',(1.83697019872103E-16,-1.,0.));
#7833=DIRECTION('center_axis',(-1.,-1.83697019872103E-16,0.));
#7834=DIRECTION('ref_axis',(1.83697019872103E-16,-1.,0.));
#7835=DIRECTION('center_axis',(-1.,-1.83697019872103E-16,0.));
#7836=DIRECTION('ref_axis',(1.83697019872103E-16,-1.,0.));
#7837=DIRECTION('',(-1.,-1.83697019872103E-16,0.));
#7838=DIRECTION('center_axis',(-1.,-1.83697019872103E-16,0.));
#7839=DIRECTION('ref_axis',(1.83697019872103E-16,-1.,0.));
#7840=DIRECTION('center_axis',(1.,1.83697019872103E-16,0.));
#7841=DIRECTION('ref_axis',(-1.83697019872103E-16,1.,0.));
#7842=DIRECTION('',(0.707106781186551,-0.707106781186544,-8.6595605623549E-17));
#7843=DIRECTION('center_axis',(-1.,-1.83697019872103E-16,0.));
#7844=DIRECTION('ref_axis',(1.83697019872103E-16,-1.,0.));
#7845=DIRECTION('center_axis',(-1.,-1.83697019872103E-16,0.));
#7846=DIRECTION('ref_axis',(1.85037170770859E-16,-1.,0.));
#7847=DIRECTION('center_axis',(-1.,-1.83697019872103E-16,0.));
#7848=DIRECTION('ref_axis',(1.83697019872103E-16,-1.,0.));
#7849=DIRECTION('center_axis',(2.24963967399279E-32,-1.22464679914735E-16,
-1.));
#7850=DIRECTION('ref_axis',(-1.85037170770859E-16,1.,-1.22464679914735E-16));
#7851=DIRECTION('center_axis',(-1.,-1.83697019872103E-16,0.));
#7852=DIRECTION('ref_axis',(1.83697019872103E-16,-1.,0.));
#7853=DIRECTION('center_axis',(-1.,-1.83697019872103E-16,0.));
#7854=DIRECTION('ref_axis',(1.83697019872103E-16,-1.,0.));
#7855=DIRECTION('center_axis',(-1.,-1.83697019872103E-16,0.));
#7856=DIRECTION('ref_axis',(1.83697019872103E-16,-1.,0.));
#7857=DIRECTION('',(1.,1.83697019872103E-16,0.));
#7858=DIRECTION('center_axis',(-1.,-1.83697019872103E-16,0.));
#7859=DIRECTION('ref_axis',(1.85037170770859E-16,-1.,0.));
#7860=DIRECTION('center_axis',(-1.,-1.83697019872103E-16,0.));
#7861=DIRECTION('ref_axis',(1.83697019872103E-16,-1.,0.));
#7862=DIRECTION('center_axis',(2.24963967399279E-32,-1.22464679914735E-16,
-1.));
#7863=DIRECTION('ref_axis',(-1.85037170770859E-16,1.,-1.22464679914735E-16));
#7864=DIRECTION('center_axis',(-1.,-1.83697019872103E-16,0.));
#7865=DIRECTION('ref_axis',(1.83697019872103E-16,-1.,0.));
#7866=DIRECTION('',(-0.707106781186551,0.707106781186544,-8.6595605623549E-17));
#7867=DIRECTION('center_axis',(-1.,-1.83697019872103E-16,0.));
#7868=DIRECTION('ref_axis',(1.83697019872103E-16,-1.,0.));
#7869=DIRECTION('center_axis',(1.,1.83697019872103E-16,0.));
#7870=DIRECTION('ref_axis',(-1.83697019872103E-16,1.,0.));
#7871=DIRECTION('center_axis',(-1.,-1.83697019872103E-16,0.));
#7872=DIRECTION('ref_axis',(1.83697019872103E-16,-1.,0.));
#7873=DIRECTION('center_axis',(1.,1.83697019872103E-16,0.));
#7874=DIRECTION('ref_axis',(-1.83697019872103E-16,1.,0.));
#7875=DIRECTION('center_axis',(-1.,-1.83697019872103E-16,0.));
#7876=DIRECTION('ref_axis',(1.83697019872103E-16,-1.,0.));
#7877=DIRECTION('center_axis',(1.,1.83697019872103E-16,0.));
#7878=DIRECTION('ref_axis',(-1.83697019872103E-16,1.,0.));
#7879=DIRECTION('center_axis',(-1.,-1.83697019872103E-16,0.));
#7880=DIRECTION('ref_axis',(1.83697019872103E-16,-1.,0.));
#7881=DIRECTION('',(-0.707106781186548,0.707106781186547,8.65956056235493E-17));
#7882=DIRECTION('center_axis',(-1.,-1.83697019872103E-16,0.));
#7883=DIRECTION('ref_axis',(1.83697019872103E-16,-1.,0.));
#7884=DIRECTION('center_axis',(-1.,-1.83697019872103E-16,0.));
#7885=DIRECTION('ref_axis',(1.83697019872103E-16,-1.,0.));
#7886=DIRECTION('center_axis',(-1.,-1.83697019872103E-16,0.));
#7887=DIRECTION('ref_axis',(1.83697019872103E-16,-1.,0.));
#7888=DIRECTION('',(1.,1.83697019872103E-16,0.));
#7889=DIRECTION('center_axis',(-1.,-1.83697019872103E-16,0.));
#7890=DIRECTION('ref_axis',(1.83697019872103E-16,-1.,0.));
#7891=DIRECTION('center_axis',(-1.,-1.83697019872103E-16,0.));
#7892=DIRECTION('ref_axis',(1.96129949112834E-16,-1.,0.));
#7893=DIRECTION('center_axis',(-2.24963967399279E-32,1.22464679914735E-16,
1.));
#7894=DIRECTION('ref_axis',(-1.63441624260695E-16,1.,-1.22464679914735E-16));
#7895=DIRECTION('center_axis',(-1.,-1.83697019872103E-16,0.));
#7896=DIRECTION('ref_axis',(1.83697019872103E-16,-1.,0.));
#7897=DIRECTION('center_axis',(-1.,-1.83697019872103E-16,0.));
#7898=DIRECTION('ref_axis',(1.83697019872103E-16,-1.,0.));
#7899=DIRECTION('center_axis',(-1.,-1.83697019872103E-16,0.));
#7900=DIRECTION('ref_axis',(1.83697019872103E-16,-1.,0.));
#7901=DIRECTION('',(1.,1.83697019872103E-16,0.));
#7902=DIRECTION('center_axis',(-1.,-1.83697019872103E-16,0.));
#7903=DIRECTION('ref_axis',(1.83697019872103E-16,-1.,0.));
#7904=DIRECTION('center_axis',(-1.,-1.83697019872103E-16,0.));
#7905=DIRECTION('ref_axis',(1.96129949112834E-16,-1.,0.));
#7906=DIRECTION('center_axis',(-1.,-1.83697019872103E-16,0.));
#7907=DIRECTION('ref_axis',(1.83697019872103E-16,-1.,0.));
#7908=DIRECTION('center_axis',(-2.24963967399279E-32,1.22464679914735E-16,
1.));
#7909=DIRECTION('ref_axis',(-1.63441624260695E-16,1.,-1.22464679914735E-16));
#7910=DIRECTION('center_axis',(-1.,-1.83697019872103E-16,0.));
#7911=DIRECTION('ref_axis',(1.83697019872103E-16,-1.,0.));
#7912=DIRECTION('center_axis',(-1.,-1.83697019872103E-16,0.));
#7913=DIRECTION('ref_axis',(1.83697019872103E-16,-1.,0.));
#7914=DIRECTION('',(1.,1.83697019872103E-16,0.));
#7915=DIRECTION('center_axis',(-1.,-1.83697019872103E-16,0.));
#7916=DIRECTION('ref_axis',(1.83697019872103E-16,-1.,0.));
#7917=DIRECTION('center_axis',(-1.,-1.83697019872103E-16,0.));
#7918=DIRECTION('ref_axis',(1.83697019872103E-16,-1.,0.));
#7919=DIRECTION('',(0.707106781186548,-0.707106781186547,8.65956056235493E-17));
#7920=DIRECTION('center_axis',(-1.,-1.83697019872103E-16,0.));
#7921=DIRECTION('ref_axis',(1.83697019872103E-16,-1.,0.));
#7922=DIRECTION('center_axis',(-1.,-1.83697019872103E-16,0.));
#7923=DIRECTION('ref_axis',(1.85037170770859E-16,-1.,0.));
#7924=DIRECTION('center_axis',(-1.,-1.83697019872103E-16,0.));
#7925=DIRECTION('ref_axis',(1.83697019872103E-16,-1.,0.));
#7926=DIRECTION('center_axis',(2.24963967399279E-32,-1.22464679914735E-16,
-1.));
#7927=DIRECTION('ref_axis',(-2.31296463463574E-16,1.,-1.22464679914735E-16));
#7928=DIRECTION('center_axis',(-1.,-1.83697019872103E-16,0.));
#7929=DIRECTION('ref_axis',(1.83697019872103E-16,-1.,0.));
#7930=DIRECTION('center_axis',(-1.,-1.83697019872103E-16,0.));
#7931=DIRECTION('ref_axis',(1.83697019872103E-16,-1.,0.));
#7932=DIRECTION('',(-1.,-1.83697019872103E-16,0.));
#7933=DIRECTION('center_axis',(-1.,-1.83697019872103E-16,0.));
#7934=DIRECTION('ref_axis',(1.83697019872103E-16,-1.,0.));
#7935=DIRECTION('center_axis',(-1.,-1.83697019872103E-16,0.));
#7936=DIRECTION('ref_axis',(1.85037170770859E-16,-1.,0.));
#7937=DIRECTION('center_axis',(2.24963967399279E-32,-1.22464679914735E-16,
-1.));
#7938=DIRECTION('ref_axis',(-2.31296463463574E-16,1.,-1.22464679914735E-16));
#7939=DIRECTION('center_axis',(-1.,-1.83697019872103E-16,0.));
#7940=DIRECTION('ref_axis',(1.83697019872103E-16,-1.,0.));
#7941=DIRECTION('center_axis',(-1.,-1.83697019872103E-16,0.));
#7942=DIRECTION('ref_axis',(1.83697019872103E-16,-1.,0.));
#7943=DIRECTION('center_axis',(-1.,-1.83697019872103E-16,0.));
#7944=DIRECTION('ref_axis',(1.83697019872103E-16,-1.,0.));
#7945=DIRECTION('center_axis',(1.,1.83697019872103E-16,0.));
#7946=DIRECTION('ref_axis',(-1.83697019872103E-16,1.,0.));
#7947=DIRECTION('center_axis',(1.,1.83697019872103E-16,0.));
#7948=DIRECTION('ref_axis',(-1.83697019872103E-16,1.,0.));
#7949=DIRECTION('center_axis',(-1.,-1.83697019872103E-16,0.));
#7950=DIRECTION('ref_axis',(1.83697019872103E-16,-1.,0.));
#7951=DIRECTION('center_axis',(-1.,-1.83697019872103E-16,0.));
#7952=DIRECTION('ref_axis',(1.83697019872103E-16,-1.,0.));
#7953=DIRECTION('',(-1.,-1.83697019872103E-16,0.));
#7954=DIRECTION('center_axis',(-1.,-1.83697019872103E-16,0.));
#7955=DIRECTION('ref_axis',(1.83697019872103E-16,-1.,0.));
#7956=DIRECTION('center_axis',(-1.,-1.83697019872103E-16,0.));
#7957=DIRECTION('ref_axis',(1.57361694361665E-16,-1.,0.));
#7958=DIRECTION('center_axis',(-1.,-1.83697019872103E-16,0.));
#7959=DIRECTION('ref_axis',(1.83697019872103E-16,-1.,0.));
#7960=DIRECTION('center_axis',(2.24963967399279E-32,-1.22464679914735E-16,
-1.));
#7961=DIRECTION('ref_axis',(-1.96702117952081E-16,1.,-1.22464679914735E-16));
#7962=DIRECTION('center_axis',(-1.,-1.83697019872103E-16,0.));
#7963=DIRECTION('ref_axis',(1.83697019872103E-16,-1.,0.));
#7964=DIRECTION('center_axis',(-1.,-1.83697019872103E-16,0.));
#7965=DIRECTION('ref_axis',(1.83697019872103E-16,-1.,0.));
#7966=DIRECTION('center_axis',(-1.,-1.83697019872103E-16,0.));
#7967=DIRECTION('ref_axis',(1.83697019872103E-16,-1.,0.));
#7968=DIRECTION('',(0.866025403784443,-0.499999999999992,6.12323399573667E-17));
#7969=DIRECTION('center_axis',(-1.,-1.83697019872103E-16,0.));
#7970=DIRECTION('ref_axis',(2.01689087919369E-16,-1.,0.));
#7971=DIRECTION('center_axis',(-1.,-1.83697019872103E-16,0.));
#7972=DIRECTION('ref_axis',(1.83697019872103E-16,-1.,0.));
#7973=DIRECTION('center_axis',(-2.24963967399279E-32,1.22464679914735E-16,
1.));
#7974=DIRECTION('ref_axis',(-1.89083519924408E-16,1.,-1.22464679914735E-16));
#7975=DIRECTION('center_axis',(-1.,-1.83697019872103E-16,0.));
#7976=DIRECTION('ref_axis',(1.88974131851091E-16,-1.,0.));
#7977=DIRECTION('center_axis',(-1.,-1.83697019872103E-16,0.));
#7978=DIRECTION('ref_axis',(1.83697019872103E-16,-1.,0.));
#7979=DIRECTION('center_axis',(-2.24963967399279E-32,1.22464679914735E-16,
1.));
#7980=DIRECTION('ref_axis',(-1.77163248610397E-16,1.,-1.22464679914735E-16));
#7981=DIRECTION('center_axis',(-1.,-1.83697019872103E-16,0.));
#7982=DIRECTION('ref_axis',(1.83697019872103E-16,-1.,0.));
#7983=DIRECTION('center_axis',(-1.,-1.83697019872103E-16,0.));
#7984=DIRECTION('ref_axis',(1.83697019872103E-16,-1.,0.));
#7985=DIRECTION('center_axis',(-1.,-1.83697019872103E-16,0.));
#7986=DIRECTION('ref_axis',(1.83697019872103E-16,-1.,0.));
#7987=DIRECTION('',(-0.500000000000007,0.866025403784435,-1.0605752387249E-16));
#7988=DIRECTION('center_axis',(-1.,-1.83697019872103E-16,0.));
#7989=DIRECTION('ref_axis',(1.91801449774277E-16,-1.,0.));
#7990=DIRECTION('center_axis',(-1.,-1.83697019872103E-16,0.));
#7991=DIRECTION('ref_axis',(1.83697019872103E-16,-1.,0.));
#7992=DIRECTION('center_axis',(-2.24963967399279E-32,1.22464679914735E-16,
1.));
#7993=DIRECTION('ref_axis',(-1.79813859163385E-16,1.,-1.22464679914735E-16));
#7994=DIRECTION('center_axis',(-1.,-1.83697019872103E-16,0.));
#7995=DIRECTION('ref_axis',(1.87747066251861E-16,-1.,0.));
#7996=DIRECTION('center_axis',(-1.,-1.83697019872103E-16,0.));
#7997=DIRECTION('ref_axis',(1.83697019872103E-16,-1.,0.));
#7998=DIRECTION('center_axis',(2.24963967399279E-32,-1.22464679914735E-16,
-1.));
#7999=DIRECTION('ref_axis',(-1.7601287461112E-16,1.,-1.22464679914735E-16));
#8000=DIRECTION('center_axis',(-1.,-1.83697019872103E-16,0.));
#8001=DIRECTION('ref_axis',(1.83697019872103E-16,-1.,0.));
#8002=DIRECTION('center_axis',(-1.,-1.83697019872103E-16,0.));
#8003=DIRECTION('ref_axis',(1.83697019872103E-16,-1.,0.));
#8004=DIRECTION('center_axis',(-1.,-1.83697019872103E-16,0.));
#8005=DIRECTION('ref_axis',(1.83697019872103E-16,-1.,0.));
#8006=DIRECTION('',(0.500000000000007,-0.866025403784435,1.0605752387249E-16));
#8007=DIRECTION('center_axis',(-1.,-1.83697019872103E-16,0.));
#8008=DIRECTION('ref_axis',(1.85037170770859E-16,-1.,0.));
#8009=DIRECTION('center_axis',(-1.,-1.83697019872103E-16,0.));
#8010=DIRECTION('ref_axis',(1.83697019872103E-16,-1.,0.));
#8011=DIRECTION('center_axis',(2.24963967399279E-32,-1.22464679914735E-16,
-1.));
#8012=DIRECTION('ref_axis',(-1.73472347597681E-16,1.,-1.22464679914735E-16));
#8013=DIRECTION('center_axis',(-1.,-1.83697019872103E-16,0.));
#8014=DIRECTION('ref_axis',(1.97210791246963E-16,-1.,0.));
#8015=DIRECTION('center_axis',(-1.,-1.83697019872103E-16,0.));
#8016=DIRECTION('ref_axis',(1.83697019872103E-16,-1.,0.));
#8017=DIRECTION('center_axis',(2.24963967399279E-32,-1.22464679914735E-16,
-1.));
#8018=DIRECTION('ref_axis',(-1.84885116794028E-16,1.,-1.22464679914735E-16));
#8019=DIRECTION('center_axis',(-1.,-1.83697019872103E-16,0.));
#8020=DIRECTION('ref_axis',(1.83697019872103E-16,-1.,0.));
#8021=DIRECTION('center_axis',(-1.,-1.83697019872103E-16,0.));
#8022=DIRECTION('ref_axis',(1.83697019872103E-16,-1.,0.));
#8023=DIRECTION('center_axis',(-1.,-1.83697019872103E-16,0.));
#8024=DIRECTION('ref_axis',(1.83697019872103E-16,-1.,0.));
#8025=DIRECTION('',(-0.866025403784443,0.499999999999992,-6.12323399573667E-17));
#8026=DIRECTION('center_axis',(1.,1.83697019872103E-16,0.));
#8027=DIRECTION('ref_axis',(-1.83697019872103E-16,1.,0.));
#8028=DIRECTION('center_axis',(1.,1.83697019872103E-16,0.));
#8029=DIRECTION('ref_axis',(-1.83697019872103E-16,1.,0.));
#8030=DIRECTION('center_axis',(-1.,-1.83697019872103E-16,0.));
#8031=DIRECTION('ref_axis',(1.83697019872103E-16,-1.,0.));
#8032=DIRECTION('center_axis',(1.,1.83697019872103E-16,0.));
#8033=DIRECTION('ref_axis',(-1.83697019872103E-16,1.,0.));
#8034=DIRECTION('center_axis',(1.,1.83697019872103E-16,0.));
#8035=DIRECTION('ref_axis',(-1.83697019872103E-16,1.,0.));
#8036=DIRECTION('center_axis',(1.,-1.83697019872103E-16,0.));
#8037=DIRECTION('ref_axis',(-1.83697019872103E-16,-1.,0.));
#8038=DIRECTION('center_axis',(-1.,1.83697019872103E-16,0.));
#8039=DIRECTION('ref_axis',(-1.83697019872103E-16,-1.,0.));
#8040=DIRECTION('',(1.,-1.83697019872103E-16,0.));
#8041=DIRECTION('center_axis',(-1.,1.83697019872103E-16,0.));
#8042=DIRECTION('ref_axis',(-1.83697019872103E-16,-1.,0.));
#8043=DIRECTION('center_axis',(1.,-1.83697019872103E-16,0.));
#8044=DIRECTION('ref_axis',(-1.57361694361665E-16,-1.,0.));
#8045=DIRECTION('center_axis',(-1.,1.83697019872103E-16,0.));
#8046=DIRECTION('ref_axis',(-1.83697019872103E-16,-1.,0.));
#8047=DIRECTION('center_axis',(-2.24963967399279E-32,-1.22464679914735E-16,
1.));
#8048=DIRECTION('ref_axis',(1.96702117952081E-16,1.,1.22464679914735E-16));
#8049=DIRECTION('center_axis',(-1.,1.83697019872103E-16,0.));
#8050=DIRECTION('ref_axis',(-1.83697019872103E-16,-1.,0.));
#8051=DIRECTION('center_axis',(1.,-1.83697019872103E-16,0.));
#8052=DIRECTION('ref_axis',(-1.83697019872103E-16,-1.,0.));
#8053=DIRECTION('center_axis',(-1.,1.83697019872103E-16,0.));
#8054=DIRECTION('ref_axis',(-1.83697019872103E-16,-1.,0.));
#8055=DIRECTION('',(-0.866025403784443,-0.499999999999992,-6.12323399573667E-17));
#8056=DIRECTION('center_axis',(1.,-1.83697019872103E-16,0.));
#8057=DIRECTION('ref_axis',(-2.01689087919369E-16,-1.,0.));
#8058=DIRECTION('center_axis',(-1.,1.83697019872103E-16,0.));
#8059=DIRECTION('ref_axis',(-1.83697019872103E-16,-1.,0.));
#8060=DIRECTION('center_axis',(2.24963967399279E-32,1.22464679914735E-16,
-1.));
#8061=DIRECTION('ref_axis',(1.89083519924408E-16,1.,1.22464679914735E-16));
#8062=DIRECTION('center_axis',(1.,-1.83697019872103E-16,0.));
#8063=DIRECTION('ref_axis',(-1.88974131851091E-16,-1.,0.));
#8064=DIRECTION('center_axis',(-1.,1.83697019872103E-16,0.));
#8065=DIRECTION('ref_axis',(-1.83697019872103E-16,-1.,0.));
#8066=DIRECTION('center_axis',(2.24963967399279E-32,1.22464679914735E-16,
-1.));
#8067=DIRECTION('ref_axis',(1.77163248610397E-16,1.,1.22464679914735E-16));
#8068=DIRECTION('center_axis',(-1.,1.83697019872103E-16,0.));
#8069=DIRECTION('ref_axis',(-1.83697019872103E-16,-1.,0.));
#8070=DIRECTION('center_axis',(1.,-1.83697019872103E-16,0.));
#8071=DIRECTION('ref_axis',(-1.83697019872103E-16,-1.,0.));
#8072=DIRECTION('center_axis',(-1.,1.83697019872103E-16,0.));
#8073=DIRECTION('ref_axis',(-1.83697019872103E-16,-1.,0.));
#8074=DIRECTION('',(0.500000000000007,0.866025403784435,1.0605752387249E-16));
#8075=DIRECTION('center_axis',(1.,-1.83697019872103E-16,0.));
#8076=DIRECTION('ref_axis',(-1.91801449774277E-16,-1.,0.));
#8077=DIRECTION('center_axis',(-1.,1.83697019872103E-16,0.));
#8078=DIRECTION('ref_axis',(-1.83697019872103E-16,-1.,0.));
#8079=DIRECTION('center_axis',(2.24963967399279E-32,1.22464679914735E-16,
-1.));
#8080=DIRECTION('ref_axis',(1.79813859163385E-16,1.,1.22464679914735E-16));
#8081=DIRECTION('center_axis',(1.,-1.83697019872103E-16,0.));
#8082=DIRECTION('ref_axis',(-1.87747066251861E-16,-1.,0.));
#8083=DIRECTION('center_axis',(-1.,1.83697019872103E-16,0.));
#8084=DIRECTION('ref_axis',(-1.83697019872103E-16,-1.,0.));
#8085=DIRECTION('center_axis',(-2.24963967399279E-32,-1.22464679914735E-16,
1.));
#8086=DIRECTION('ref_axis',(1.7601287461112E-16,1.,1.22464679914735E-16));
#8087=DIRECTION('center_axis',(-1.,1.83697019872103E-16,0.));
#8088=DIRECTION('ref_axis',(-1.83697019872103E-16,-1.,0.));
#8089=DIRECTION('center_axis',(1.,-1.83697019872103E-16,0.));
#8090=DIRECTION('ref_axis',(-1.83697019872103E-16,-1.,0.));
#8091=DIRECTION('center_axis',(-1.,1.83697019872103E-16,0.));
#8092=DIRECTION('ref_axis',(-1.83697019872103E-16,-1.,0.));
#8093=DIRECTION('',(-0.500000000000007,-0.866025403784435,-1.0605752387249E-16));
#8094=DIRECTION('center_axis',(1.,-1.83697019872103E-16,0.));
#8095=DIRECTION('ref_axis',(-1.85037170770859E-16,-1.,0.));
#8096=DIRECTION('center_axis',(-1.,1.83697019872103E-16,0.));
#8097=DIRECTION('ref_axis',(-1.83697019872103E-16,-1.,0.));
#8098=DIRECTION('center_axis',(-2.24963967399279E-32,-1.22464679914735E-16,
1.));
#8099=DIRECTION('ref_axis',(1.73472347597681E-16,1.,1.22464679914735E-16));
#8100=DIRECTION('center_axis',(1.,-1.83697019872103E-16,0.));
#8101=DIRECTION('ref_axis',(-1.97210791246963E-16,-1.,0.));
#8102=DIRECTION('center_axis',(-1.,1.83697019872103E-16,0.));
#8103=DIRECTION('ref_axis',(-1.83697019872103E-16,-1.,0.));
#8104=DIRECTION('center_axis',(-2.24963967399279E-32,-1.22464679914735E-16,
1.));
#8105=DIRECTION('ref_axis',(1.84885116794028E-16,1.,1.22464679914735E-16));
#8106=DIRECTION('center_axis',(-1.,1.83697019872103E-16,0.));
#8107=DIRECTION('ref_axis',(-1.83697019872103E-16,-1.,0.));
#8108=DIRECTION('center_axis',(1.,-1.83697019872103E-16,0.));
#8109=DIRECTION('ref_axis',(-1.83697019872103E-16,-1.,0.));
#8110=DIRECTION('center_axis',(-1.,1.83697019872103E-16,0.));
#8111=DIRECTION('ref_axis',(-1.83697019872103E-16,-1.,0.));
#8112=DIRECTION('',(0.866025403784443,0.499999999999992,6.12323399573667E-17));
#8113=DIRECTION('center_axis',(-1.,1.83697019872103E-16,0.));
#8114=DIRECTION('ref_axis',(1.83697019872103E-16,1.,0.));
#8115=DIRECTION('center_axis',(-1.,1.83697019872103E-16,0.));
#8116=DIRECTION('ref_axis',(1.83697019872103E-16,1.,0.));
#8117=DIRECTION('center_axis',(1.,-1.83697019872103E-16,0.));
#8118=DIRECTION('ref_axis',(-1.83697019872103E-16,-1.,0.));
#8119=DIRECTION('center_axis',(-1.,1.83697019872103E-16,0.));
#8120=DIRECTION('ref_axis',(1.83697019872103E-16,1.,0.));
#8121=DIRECTION('center_axis',(-1.,1.83697019872103E-16,0.));
#8122=DIRECTION('ref_axis',(1.83697019872103E-16,1.,0.));
#9637=CARTESIAN_POINT('',(0.,0.,0.));
#9638=CARTESIAN_POINT('Origin',(-1.8,0.,0.));
#9639=CARTESIAN_POINT('',(-1.7,4.8,-5.8783046359073E-16));
#9640=CARTESIAN_POINT('Origin',(-1.7,1.83697019872105E-17,0.));
#9641=CARTESIAN_POINT('',(-1.955,4.8,-5.8783046359073E-16));
#9642=CARTESIAN_POINT('',(-1.8,4.8,-5.87830463590729E-16));
#9643=CARTESIAN_POINT('Origin',(-1.955,-2.84730380801758E-17,0.));
#9644=CARTESIAN_POINT('Origin',(-1.8,0.,0.));
#9645=CARTESIAN_POINT('',(1.7,4.872,-5.96647920544591E-16));
#9646=CARTESIAN_POINT('Origin',(1.7,6.42939569552361E-16,0.));
#9647=CARTESIAN_POINT('',(-1.7,4.872,-5.96647920544591E-16));
#9648=CARTESIAN_POINT('',(-1.8,4.872,-5.96647920544591E-16));
#9649=CARTESIAN_POINT('Origin',(-1.7,1.83697019872105E-17,0.));
#9650=CARTESIAN_POINT('Origin',(-1.8,0.,0.));
#9651=CARTESIAN_POINT('',(1.955,-4.8,5.90585918888811E-16));
#9652=CARTESIAN_POINT('',(1.955,4.8,-5.87830463590729E-16));
#9653=CARTESIAN_POINT('Origin',(1.955,6.89782309619747E-16,0.));
#9654=CARTESIAN_POINT('Origin',(1.955,6.89782309619747E-16,0.));
#9655=CARTESIAN_POINT('',(1.7,4.8,-5.87830463590729E-16));
#9656=CARTESIAN_POINT('',(-1.8,4.8,-5.87830463590729E-16));
#9657=CARTESIAN_POINT('Origin',(1.7,6.42939569552361E-16,0.));
#9658=CARTESIAN_POINT('Origin',(1.955,6.89782309619747E-16,0.));
#9659=CARTESIAN_POINT('',(2.,-4.845,-5.93341374186893E-16));
#9660=CARTESIAN_POINT('',(1.955,-4.8,-5.87830463590729E-16));
#9661=CARTESIAN_POINT('Origin',(2.,6.98048675513991E-16,0.));
#9662=CARTESIAN_POINT('Origin',(1.8,8.67361737988404E-16,0.));
#9663=CARTESIAN_POINT('',(1.8,6.,-7.34788079488412E-16));
#9664=CARTESIAN_POINT('Origin',(1.8,6.61309271539571E-16,0.));
#9665=CARTESIAN_POINT('',(2.,5.8,-7.10295143505465E-16));
#9666=CARTESIAN_POINT('Origin',(1.8,5.8,-7.10295143505465E-16));
#9667=CARTESIAN_POINT('Origin',(2.,6.98048675513991E-16,0.));
#9668=CARTESIAN_POINT('Origin',(-1.8,0.,0.));
#9669=CARTESIAN_POINT('',(-1.8,6.,-7.34788079488412E-16));
#9670=CARTESIAN_POINT('Origin',(-1.8,2.02467570659351E-31,0.));
#9671=CARTESIAN_POINT('',(-1.8,6.,-7.34788079488412E-16));
#9672=CARTESIAN_POINT('Origin',(-1.8,0.,0.));
#9673=CARTESIAN_POINT('',(-2.,5.8,-7.10295143505465E-16));
#9674=CARTESIAN_POINT('Origin',(-2.,-3.67394039744204E-17,0.));
#9675=CARTESIAN_POINT('Origin',(-1.8,5.8,-7.10295143505465E-16));
#9676=CARTESIAN_POINT('Origin',(-2.,-3.67394039744204E-17,0.));
#9677=CARTESIAN_POINT('',(-2.,4.845,-5.93341374186893E-16));
#9678=CARTESIAN_POINT('',(-2.,4.845,-5.93341374186893E-16));
#9679=CARTESIAN_POINT('Origin',(-2.,-3.67394039744204E-17,0.));
#9680=CARTESIAN_POINT('Origin',(-2.,5.8,0.));
#9681=CARTESIAN_POINT('Origin',(2.,5.8,0.));
#9682=CARTESIAN_POINT('Origin',(1.7,4.8,0.));
#9683=CARTESIAN_POINT('Origin',(-1.7,4.8,0.));
#9684=CARTESIAN_POINT('Origin',(-1.955,-2.84730380801757E-17,0.));
#9685=CARTESIAN_POINT('',(-1.955,3.1184375,3.81898450271607E-16));
#9686=CARTESIAN_POINT('',(-1.955,-3.1184375,-3.81898450271607E-16));
#9687=CARTESIAN_POINT('Origin',(-1.955,-2.84730380801757E-17,0.));
#9688=CARTESIAN_POINT('',(-2.,-3.0734375,-3.76387539675444E-16));
#9689=CARTESIAN_POINT('',(-1.955,-3.1184375,-3.81898450271607E-16));
#9690=CARTESIAN_POINT('Origin',(-2.,-3.67394039744204E-17,0.));
#9691=CARTESIAN_POINT('Origin',(-1.955,-2.84730380801757E-17,0.));
#9692=CARTESIAN_POINT('Origin',(-1.8,0.,0.));
#9693=CARTESIAN_POINT('',(-1.7890625,3.1184375,-3.81898450271607E-16));
#9694=CARTESIAN_POINT('',(-1.8,3.1184375,-3.81898450271607E-16));
#9695=CARTESIAN_POINT('Origin',(-1.7890625,2.00918615485137E-18,0.));
#9696=CARTESIAN_POINT('Origin',(-1.7890625,0.,0.));
#9697=CARTESIAN_POINT('',(-1.6625,3.2,-3.91886975727153E-16));
#9698=CARTESIAN_POINT('Origin',(-1.7890625,3.25741379310345,-3.98918137522258E-16));
#9699=CARTESIAN_POINT('Origin',(-1.6625,2.52583402324144E-17,0.));
#9700=CARTESIAN_POINT('Origin',(-1.8,0.,0.));
#9701=CARTESIAN_POINT('',(-1.6625,3.272,-4.00704432681014E-16));
#9702=CARTESIAN_POINT('Origin',(-1.6625,2.52583402324144E-17,0.));
#9703=CARTESIAN_POINT('',(1.6625,3.272,-4.00704432681014E-16));
#9704=CARTESIAN_POINT('',(-1.8,3.272,-4.00704432681014E-16));
#9705=CARTESIAN_POINT('Origin',(1.6625,6.36050931307157E-16,0.));
#9706=CARTESIAN_POINT('Origin',(1.7890625,8.67361737988404E-16,0.));
#9707=CARTESIAN_POINT('',(1.6625,3.2,-3.91886975727153E-16));
#9708=CARTESIAN_POINT('Origin',(1.6625,6.36050931307157E-16,0.));
#9709=CARTESIAN_POINT('',(1.7890625,3.1184375,-3.81898450271607E-16));
#9710=CARTESIAN_POINT('Origin',(1.7890625,3.25741379310345,-3.98918137522258E-16));
#9711=CARTESIAN_POINT('Origin',(1.7890625,6.5930008538472E-16,0.));
#9712=CARTESIAN_POINT('Origin',(-1.8,0.,0.));
#9713=CARTESIAN_POINT('',(1.955,3.1184375,-3.81898450271607E-16));
#9714=CARTESIAN_POINT('',(-1.8,3.1184375,-3.81898450271607E-16));
#9715=CARTESIAN_POINT('Origin',(1.955,6.89782309619747E-16,0.));
#9716=CARTESIAN_POINT('Origin',(2.,6.98048675513991E-16,0.));
#9717=CARTESIAN_POINT('',(2.,3.0734375,-3.76387539675444E-16));
#9718=CARTESIAN_POINT('',(2.,3.0734375,-3.76387539675444E-16));
#9719=CARTESIAN_POINT('Origin',(2.,6.98048675513991E-16,0.));
#9720=CARTESIAN_POINT('Origin',(1.8,8.67361737988404E-16,0.));
#9721=CARTESIAN_POINT('',(2.,2.2,-2.69422295812418E-16));
#9722=CARTESIAN_POINT('Origin',(2.,6.98048675513991E-16,0.));
#9723=CARTESIAN_POINT('',(1.8,2.,-2.44929359829471E-16));
#9724=CARTESIAN_POINT('Origin',(1.8,2.2,-2.69422295812418E-16));
#9725=CARTESIAN_POINT('Origin',(1.8,6.61309271539571E-16,0.));
#9726=CARTESIAN_POINT('Origin',(-1.8,0.,0.));
#9727=CARTESIAN_POINT('',(-1.8,2.,-2.44929359829471E-16));
#9728=CARTESIAN_POINT('',(-1.8,2.,-2.44929359829471E-16));
#9729=CARTESIAN_POINT('Origin',(-1.8,1.86988015034452E-31,0.));
#9730=CARTESIAN_POINT('Origin',(-1.8,0.,0.));
#9731=CARTESIAN_POINT('',(-2.,2.2,-2.69422295812418E-16));
#9732=CARTESIAN_POINT('Origin',(-1.8,2.2,-2.69422295812418E-16));
#9733=CARTESIAN_POINT('Origin',(-2.,-3.67394039744205E-17,0.));
#9734=CARTESIAN_POINT('Origin',(2.,2.2,0.));
#9735=CARTESIAN_POINT('Origin',(1.6625,3.272,0.));
#9736=CARTESIAN_POINT('Origin',(-1.6625,3.2,0.));
#9737=CARTESIAN_POINT('Origin',(-2.,2.2,0.));
#9738=CARTESIAN_POINT('Origin',(-1.8,0.,0.));
#9739=CARTESIAN_POINT('',(1.95,3.2,-3.91886975727153E-16));
#9740=CARTESIAN_POINT('Origin',(1.95,6.88863824520387E-16,0.));
#9741=CARTESIAN_POINT('',(1.85,3.2,-3.91886975727153E-16));
#9742=CARTESIAN_POINT('',(-1.8,3.2,-3.91886975727153E-16));
#9743=CARTESIAN_POINT('Origin',(1.85,6.70494122533176E-16,0.));
#9744=CARTESIAN_POINT('Origin',(1.86,8.67361737988404E-16,0.));
#9745=CARTESIAN_POINT('',(1.905,4.22108058265378,-5.16933282449E-16));
#9746=CARTESIAN_POINT('Origin',(1.905,6.80597458626142E-16,0.));
#9747=CARTESIAN_POINT('',(1.95,4.14313829631318,-5.07388105300476E-16));
#9748=CARTESIAN_POINT('Origin',(1.86,4.14313829631318,-5.07388105300475E-16));
#9749=CARTESIAN_POINT('Origin',(1.95,6.88863824520387E-16,0.));
#9750=CARTESIAN_POINT('Origin',(1.65333333333334,6.34367041958329E-16,0.));
#9751=CARTESIAN_POINT('',(1.65333333333334,4.36638040039984,-5.3472737812094E-16));
#9752=CARTESIAN_POINT('Origin',(1.65333333333334,6.34367041958329E-16,0.));
#9753=CARTESIAN_POINT('',(1.65333333333334,4.36638040039984,-5.3472737812094E-16));
#9754=CARTESIAN_POINT('Origin',(1.66333333333334,8.67361737988404E-16,0.));
#9755=CARTESIAN_POINT('',(1.64333333333333,4.38370090847553,-5.3684852859839E-16));
#9756=CARTESIAN_POINT('Origin',(1.64333333333334,6.32530071759608E-16,0.));
#9757=CARTESIAN_POINT('Origin',(1.66333333333334,4.38370090847553,-5.3684852859839E-16));
#9758=CARTESIAN_POINT('Origin',(1.76333333333333,8.67361737988404E-16,0.));
#9759=CARTESIAN_POINT('',(1.86725638178747,4.64,-5.68236114804372E-16));
#9760=CARTESIAN_POINT('Origin',(1.86725638178747,6.73664068441309E-16,0.));
#9761=CARTESIAN_POINT('',(1.64333333333333,4.58,-5.60888234009488E-16));
#9762=CARTESIAN_POINT('Origin',(1.76333333333333,4.58,-5.60888234009488E-16));
#9763=CARTESIAN_POINT('Origin',(1.64333333333334,6.32530071759608E-16,0.));
#9764=CARTESIAN_POINT('Origin',(1.90725638178747,6.81011949236193E-16,0.));
#9765=CARTESIAN_POINT('',(1.90725638178747,4.57071796769724,-5.59751512894572E-16));
#9766=CARTESIAN_POINT('Origin',(1.90725638178747,6.81011949236193E-16,0.));
#9767=CARTESIAN_POINT('',(1.90725638178747,4.57071796769724,-5.59751512894572E-16));
#9768=CARTESIAN_POINT('Origin',(1.80333333333334,8.67361737988404E-16,0.));
#9769=CARTESIAN_POINT('',(1.80333333333334,4.39071796769724,-5.3770787050992E-16));
#9770=CARTESIAN_POINT('Origin',(1.80333333333334,6.61921594939145E-16,0.));
#9771=CARTESIAN_POINT('Origin',(1.80333333333334,4.51071796769724,-5.52403632099688E-16));
#9772=CARTESIAN_POINT('Origin',(1.80333333333334,8.67361737988404E-16,0.));
#9773=CARTESIAN_POINT('',(1.99385892216591,4.62071796769724,-5.65874746890309E-16));
#9774=CARTESIAN_POINT('Origin',(1.99385892216591,6.96920577817067E-16,0.));
#9775=CARTESIAN_POINT('',(1.80333333333334,4.29071796769724,-5.25461402518447E-16));
#9776=CARTESIAN_POINT('Origin',(1.80333333333334,4.51071796769724,-5.52403632099688E-16));
#9777=CARTESIAN_POINT('Origin',(1.80333333333334,6.61921594939145E-16,0.));
#9778=CARTESIAN_POINT('Origin',(1.99385892216591,6.96920577817067E-16,0.));
#9779=CARTESIAN_POINT('',(1.95385892216591,4.69,-5.74359348800109E-16));
#9780=CARTESIAN_POINT('Origin',(1.95385892216591,6.89572697022182E-16,0.));
#9781=CARTESIAN_POINT('',(1.99385892216591,4.62071796769724,-5.65874746890309E-16));
#9782=CARTESIAN_POINT('Origin',(1.76333333333333,8.67361737988404E-16,0.));
#9783=CARTESIAN_POINT('',(1.54333333333334,4.58,-5.60888234009488E-16));
#9784=CARTESIAN_POINT('Origin',(1.54333333333334,6.14160369772398E-16,0.));
#9785=CARTESIAN_POINT('Origin',(1.76333333333333,4.58,-5.60888234009488E-16));
#9786=CARTESIAN_POINT('Origin',(1.66333333333334,8.67361737988404E-16,0.));
#9787=CARTESIAN_POINT('',(1.60333333333334,4.27977786002139,-5.24121625733691E-16));
#9788=CARTESIAN_POINT('Origin',(1.60333333333334,6.25182190964724E-16,0.));
#9789=CARTESIAN_POINT('',(1.54333333333333,4.38370090847553,-5.3684852859839E-16));
#9790=CARTESIAN_POINT('Origin',(1.66333333333334,4.38370090847553,-5.3684852859839E-16));
#9791=CARTESIAN_POINT('Origin',(1.54333333333334,6.14160369772398E-16,0.));
#9792=CARTESIAN_POINT('Origin',(1.60333333333334,6.25182190964724E-16,0.));
#9793=CARTESIAN_POINT('',(1.85,4.13736479362129,-5.06681055141326E-16));
#9794=CARTESIAN_POINT('Origin',(1.85,6.70494122533176E-16,0.));
#9795=CARTESIAN_POINT('',(1.60333333333334,4.27977786002139,-5.2412162573369E-16));
#9796=CARTESIAN_POINT('Origin',(1.85,4.14313829631318,0.));
#9797=CARTESIAN_POINT('Origin',(1.54333333333334,4.58,0.));
#9798=CARTESIAN_POINT('Origin',(1.80333333333334,4.29071796769724,0.));
#9799=CARTESIAN_POINT('Origin',(1.64333333333334,4.58,0.));
#9800=CARTESIAN_POINT('Origin',(1.95,4.14313829631318,0.));
#9801=CARTESIAN_POINT('Origin',(1.8,0.,0.));
#9802=CARTESIAN_POINT('',(-1.95,3.2,3.91886975727153E-16));
#9803=CARTESIAN_POINT('Origin',(-1.95,6.88863824520387E-16,0.));
#9804=CARTESIAN_POINT('',(-1.85,3.2,3.91886975727153E-16));
#9805=CARTESIAN_POINT('',(1.8,3.2,3.91886975727153E-16));
#9806=CARTESIAN_POINT('Origin',(-1.85,6.70494122533176E-16,0.));
#9807=CARTESIAN_POINT('Origin',(-1.86,8.67361737988404E-16,0.));
#9808=CARTESIAN_POINT('',(-1.905,4.22108058265378,5.16933282449E-16));
#9809=CARTESIAN_POINT('Origin',(-1.905,6.80597458626142E-16,0.));
#9810=CARTESIAN_POINT('',(-1.95,4.14313829631318,5.07388105300476E-16));
#9811=CARTESIAN_POINT('Origin',(-1.86,4.14313829631318,5.07388105300475E-16));
#9812=CARTESIAN_POINT('Origin',(-1.95,6.88863824520387E-16,0.));
#9813=CARTESIAN_POINT('Origin',(-1.65333333333334,6.34367041958329E-16,
0.));
#9814=CARTESIAN_POINT('',(-1.65333333333334,4.36638040039984,5.3472737812094E-16));
#9815=CARTESIAN_POINT('Origin',(-1.65333333333334,6.34367041958329E-16,
0.));
#9816=CARTESIAN_POINT('',(-1.65333333333334,4.36638040039984,5.3472737812094E-16));
#9817=CARTESIAN_POINT('Origin',(-1.66333333333334,8.67361737988404E-16,
0.));
#9818=CARTESIAN_POINT('',(-1.64333333333333,4.38370090847553,5.3684852859839E-16));
#9819=CARTESIAN_POINT('Origin',(-1.64333333333334,6.32530071759608E-16,
0.));
#9820=CARTESIAN_POINT('Origin',(-1.66333333333334,4.38370090847553,5.3684852859839E-16));
#9821=CARTESIAN_POINT('Origin',(-1.76333333333333,8.67361737988404E-16,
0.));
#9822=CARTESIAN_POINT('',(-1.86725638178747,4.64,5.68236114804372E-16));
#9823=CARTESIAN_POINT('Origin',(-1.86725638178747,6.73664068441309E-16,
0.));
#9824=CARTESIAN_POINT('',(-1.64333333333333,4.58,5.60888234009488E-16));
#9825=CARTESIAN_POINT('Origin',(-1.76333333333333,4.58,5.60888234009488E-16));
#9826=CARTESIAN_POINT('Origin',(-1.64333333333334,6.32530071759608E-16,
0.));
#9827=CARTESIAN_POINT('Origin',(-1.90725638178747,6.81011949236193E-16,
0.));
#9828=CARTESIAN_POINT('',(-1.90725638178747,4.57071796769724,5.59751512894572E-16));
#9829=CARTESIAN_POINT('Origin',(-1.90725638178747,6.81011949236193E-16,
0.));
#9830=CARTESIAN_POINT('',(-1.90725638178747,4.57071796769724,5.59751512894572E-16));
#9831=CARTESIAN_POINT('Origin',(-1.80333333333334,8.67361737988404E-16,
0.));
#9832=CARTESIAN_POINT('',(-1.80333333333334,4.39071796769724,5.3770787050992E-16));
#9833=CARTESIAN_POINT('Origin',(-1.80333333333334,6.61921594939145E-16,
0.));
#9834=CARTESIAN_POINT('Origin',(-1.80333333333334,4.51071796769724,5.52403632099688E-16));
#9835=CARTESIAN_POINT('Origin',(-1.80333333333334,8.67361737988404E-16,
0.));
#9836=CARTESIAN_POINT('',(-1.99385892216591,4.62071796769724,5.65874746890309E-16));
#9837=CARTESIAN_POINT('Origin',(-1.99385892216591,6.96920577817067E-16,
0.));
#9838=CARTESIAN_POINT('',(-1.80333333333334,4.29071796769724,5.25461402518447E-16));
#9839=CARTESIAN_POINT('Origin',(-1.80333333333334,4.51071796769724,5.52403632099688E-16));
#9840=CARTESIAN_POINT('Origin',(-1.80333333333334,6.61921594939145E-16,
0.));
#9841=CARTESIAN_POINT('Origin',(-1.99385892216591,6.96920577817067E-16,
0.));
#9842=CARTESIAN_POINT('',(-1.95385892216591,4.69,5.74359348800109E-16));
#9843=CARTESIAN_POINT('Origin',(-1.95385892216591,6.89572697022182E-16,
0.));
#9844=CARTESIAN_POINT('',(-1.99385892216591,4.62071796769724,5.65874746890309E-16));
#9845=CARTESIAN_POINT('Origin',(-1.76333333333333,8.67361737988404E-16,
0.));
#9846=CARTESIAN_POINT('',(-1.54333333333334,4.58,5.60888234009488E-16));
#9847=CARTESIAN_POINT('Origin',(-1.54333333333334,6.14160369772398E-16,
0.));
#9848=CARTESIAN_POINT('Origin',(-1.76333333333333,4.58,5.60888234009488E-16));
#9849=CARTESIAN_POINT('Origin',(-1.66333333333334,8.67361737988404E-16,
0.));
#9850=CARTESIAN_POINT('',(-1.60333333333334,4.27977786002139,5.24121625733691E-16));
#9851=CARTESIAN_POINT('Origin',(-1.60333333333334,6.25182190964724E-16,
0.));
#9852=CARTESIAN_POINT('',(-1.54333333333333,4.38370090847553,5.3684852859839E-16));
#9853=CARTESIAN_POINT('Origin',(-1.66333333333334,4.38370090847553,5.3684852859839E-16));
#9854=CARTESIAN_POINT('Origin',(-1.54333333333334,6.14160369772398E-16,
0.));
#9855=CARTESIAN_POINT('Origin',(-1.60333333333334,6.25182190964724E-16,
0.));
#9856=CARTESIAN_POINT('',(-1.85,4.13736479362129,5.06681055141326E-16));
#9857=CARTESIAN_POINT('Origin',(-1.85,6.70494122533176E-16,0.));
#9858=CARTESIAN_POINT('',(-1.60333333333334,4.27977786002139,5.2412162573369E-16));
#9859=CARTESIAN_POINT('Origin',(-1.85,4.14313829631318,0.));
#9860=CARTESIAN_POINT('Origin',(-1.54333333333334,4.58,0.));
#9861=CARTESIAN_POINT('Origin',(-1.80333333333334,4.29071796769724,0.));
#9862=CARTESIAN_POINT('Origin',(-1.64333333333334,4.58,0.));
#9863=CARTESIAN_POINT('Origin',(-1.95,4.14313829631318,0.));
#9880=UNCERTAINTY_MEASURE_WITH_UNIT(LENGTH_MEASURE(0.01),#9892,
'DISTANCE_ACCURACY_VALUE',
'Maximum model space distance between geometric entities at asserted c
onnectivities');
#9881=UNCERTAINTY_MEASURE_WITH_UNIT(LENGTH_MEASURE(0.01),#9892,
'DISTANCE_ACCURACY_VALUE',
'Maximum model space distance between geometric entities at asserted c
onnectivities');
#9890=(
GEOMETRIC_REPRESENTATION_CONTEXT(3)
GLOBAL_UNCERTAINTY_ASSIGNED_CONTEXT((#9880))
GLOBAL_UNIT_ASSIGNED_CONTEXT((#9892,#9894,#9895))
REPRESENTATION_CONTEXT('','3D')
);
#9891=(
GEOMETRIC_REPRESENTATION_CONTEXT(3)
GLOBAL_UNCERTAINTY_ASSIGNED_CONTEXT((#9881))
GLOBAL_UNIT_ASSIGNED_CONTEXT((#9892,#9894,#9895))
REPRESENTATION_CONTEXT('','3D')
);
#9892=(
LENGTH_UNIT()
NAMED_UNIT(*)
SI_UNIT(.MILLI.,.METRE.)
);
#9894=(
NAMED_UNIT(*)
PLANE_ANGLE_UNIT()
SI_UNIT($,.RADIAN.)
);
#9895=(
NAMED_UNIT(*)
SI_UNIT($,.STERADIAN.)
SOLID_ANGLE_UNIT()
);
#9904=SHAPE_DEFINITION_REPRESENTATION(#9913,#9930);
#9913=PRODUCT_DEFINITION_SHAPE('',$,#9940);
#9930=SHAPE_REPRESENTATION('',(#6220),#9890);
#9931=PRODUCT_DEFINITION_CONTEXT('part definition',#9960,'design');
#9940=PRODUCT_DEFINITION(
'7804K102_Corrosion-Resistant 440C Stainless Steel Ball Bearing_1',
'Bearing_02',#9949,#9931);
#9949=PRODUCT_DEFINITION_FORMATION('',$,#9970);
#9960=APPLICATION_CONTEXT(
'Core Data for Automotive Mechanical Design Process');
#9961=PRODUCT_CONTEXT('part definition',#9960,'mechanical');
#9970=PRODUCT(
'7804K102_Corrosion-Resistant 440C Stainless Steel Ball Bearing_1',
'Bearing_02',$,(#9961));
#9972=PRESENTATION_STYLE_ASSIGNMENT((#9977));
#9977=SURFACE_STYLE_USAGE(.BOTH.,#9982);
#9982=SURFACE_SIDE_STYLE('',(#9987));
#9987=SURFACE_STYLE_FILL_AREA(#9992);
#9992=FILL_AREA_STYLE('Opaque(160,160,160)',(#9997));
#9997=FILL_AREA_STYLE_COLOUR('Opaque(160,160,160)',#10002);
#10002=COLOUR_RGB('Opaque(160,160,160)', 0.09019608, 0.27058824, 0.51372549);
ENDSEC;
END-ISO-10303-21;
